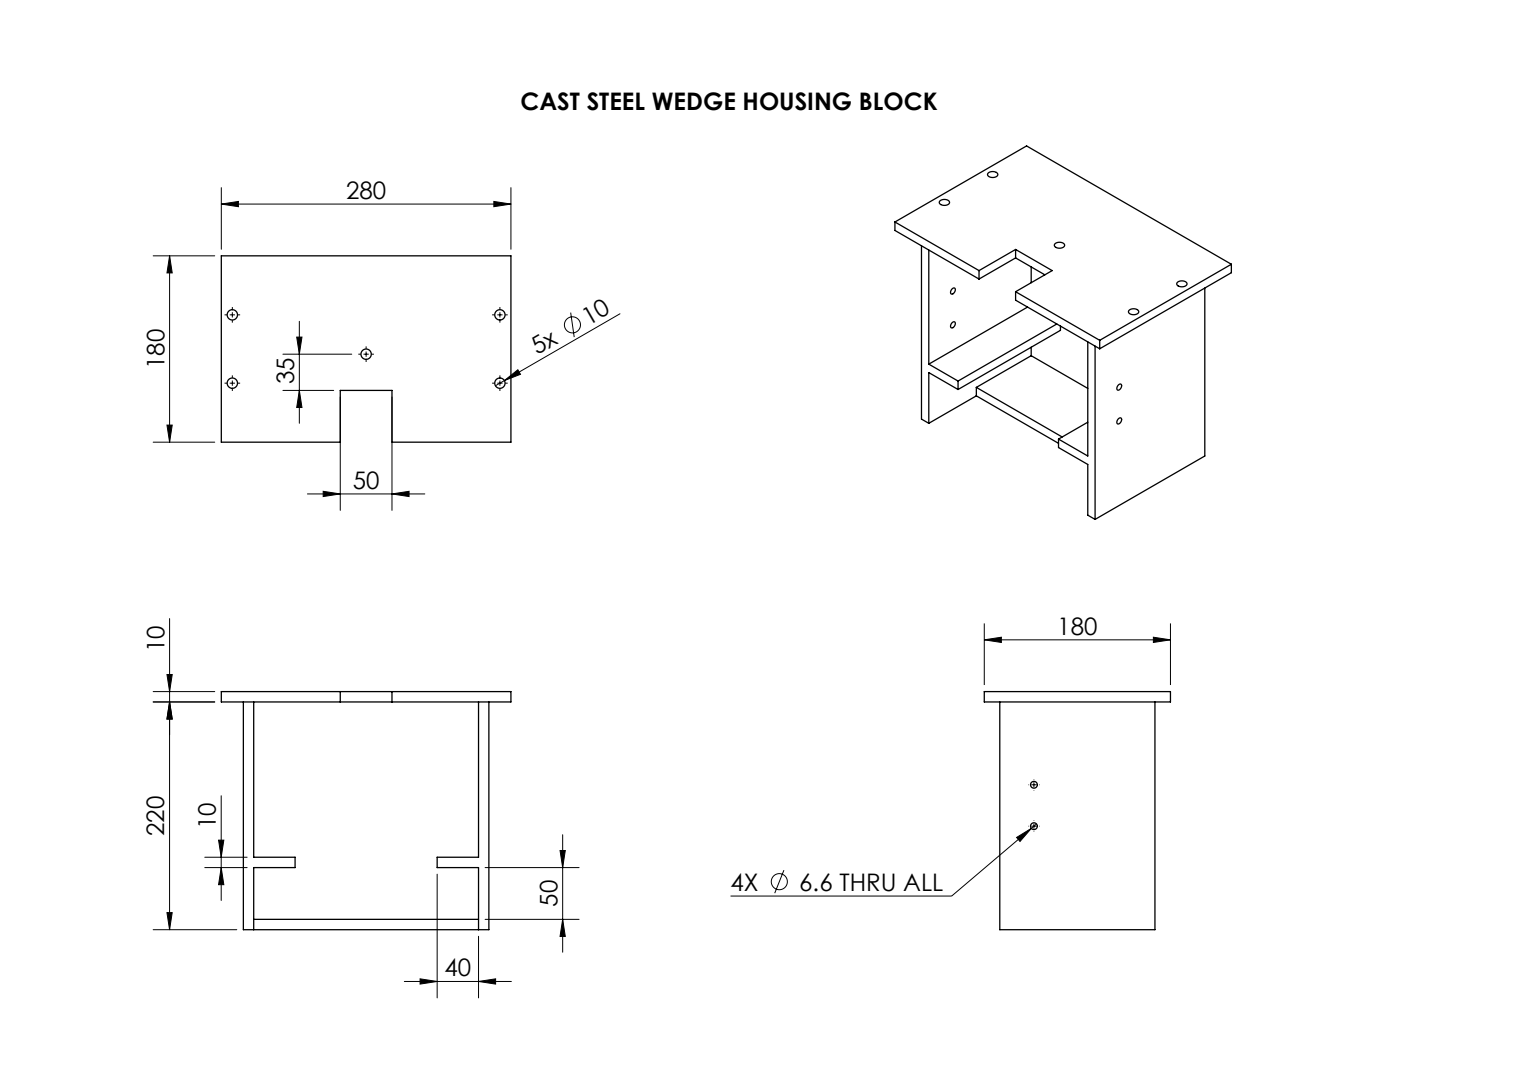
ISO-10303-21;
HEADER;
FILE_DESCRIPTION (('STEP AP214'),
    '1' );
FILE_NAME ('Cast Steel Wedge Housing Block.step',
    '2026-09-24T10:26:00',
    ( '' ),
    ( '' ),
    'SwSTEP 2.0',
    'SolidWorks 2026',
    '' );
FILE_SCHEMA (( 'AUTOMOTIVE_DESIGN' ));
ENDSEC;

DATA;
#1=VERTEX_POINT ( 'NONE', #3163 ) ;
#16=LINE ( 'NONE', #8451, #3074 ) ;
#26=LINE ( 'NONE', #9828, #8340 ) ;
#37=EDGE_CURVE ( 'NONE', #1523, #9034, #1990, .T. ) ;
#49=CARTESIAN_POINT ( 'NONE',  ( -129.3408537872145132, 199.5765550933606107, -75.00000000000001421 ) ) ;
#82=CARTESIAN_POINT ( 'NONE',  ( -108.6817075744281595, 69.57655509336026967, 0.000000000000000000 ) ) ;
#105=ORIENTED_EDGE ( 'NONE', *, *, #7029, .T. ) ;
#112=ORIENTED_EDGE ( 'NONE', *, *, #12518, .T. ) ;
#115=LINE ( 'NONE', #14321, #13122 ) ;
#130=EDGE_CURVE ( 'NONE', #3893, #6812, #6927, .T. ) ;
#149=LINE ( 'NONE', #2412, #13592 ) ;
#167=CARTESIAN_POINT ( 'NONE',  ( 0.000000000000000000, 0.000000000000000000, 0.000000000000000000 ) ) ;
#179=( NAMED_UNIT ( * ) PLANE_ANGLE_UNIT ( ) SI_UNIT ( $, .RADIAN. ) );
#185=ORIENTED_EDGE ( 'NONE', *, *, #3525, .T. ) ;
#186=DIRECTION ( 'NONE',  ( 0.000000000000000000, 0.000000000000000000, -1.000000000000000000 ) ) ;
#191=FACE_OUTER_BOUND ( 'NONE', #2606, .T. ) ;
#195=ADVANCED_FACE ( 'NONE', ( #8392 ), #5103, .F. ) ;
#215=LINE ( 'NONE', #3596, #1161 ) ;
#225=EDGE_CURVE ( 'NONE', #10568, #2459, #4887, .T. ) ;
#236=DIRECTION ( 'NONE',  ( 1.000000000000000000, -0.000000000000000000, -0.000000000000000000 ) ) ;
#237=AXIS2_PLACEMENT_3D ( 'NONE', #9091, #4649, #3762 ) ;
#243=DIRECTION ( 'NONE',  ( 1.000000000000000000, 1.723842398015259277E-15, 0.000000000000000000 ) ) ;
#250=PRESENTATION_STYLE_ASSIGNMENT (( #7854 ) ) ;
#252=LINE ( 'NONE', #13664, #5773 ) ;
#254=VERTEX_POINT ( 'NONE', #10524 ) ;
#256=ORIENTED_EDGE ( 'NONE', *, *, #409, .F. ) ;
#264=ADVANCED_FACE ( 'NONE', ( #14056 ), #3951, .T. ) ;
#268=CIRCLE ( 'NONE', #9369, 5.000000000000004441 ) ;
#275=FILL_AREA_STYLE_COLOUR ( '', #447 ) ;
#287=AXIS2_PLACEMENT_3D ( 'NONE', #9499, #13966, #10597 ) ;
#300=DIRECTION ( 'NONE',  ( -1.000000000000000000, -1.276920294826118092E-16, 0.000000000000000000 ) ) ;
#333=CARTESIAN_POINT ( 'NONE',  ( 108.6817075744280174, -30.42344490663958112, 33.00000000000002842 ) ) ;
#334=LINE ( 'NONE', #480, #12683 ) ;
#335=ORIENTED_EDGE ( 'NONE', *, *, #3874, .F. ) ;
#347=PRESENTATION_STYLE_ASSIGNMENT (( #11533 ) ) ;
#352=CARTESIAN_POINT ( 'NONE',  ( 25.00000000000000000, 189.5765550933606107, 47.99999999999998579 ) ) ;
#365=CARTESIAN_POINT ( 'NONE',  ( 129.3408537872138595, 189.5765550933606107, -4.000000000000019540 ) ) ;
#380=DIRECTION ( 'NONE',  ( 0.000000000000000000, 0.000000000000000000, -1.000000000000000000 ) ) ;
#393=ORIENTED_EDGE ( 'NONE', *, *, #4064, .F. ) ;
#408=VERTEX_POINT ( 'NONE', #8758 ) ;
#409=EDGE_CURVE ( 'NONE', #3034, #3463, #1002, .T. ) ;
#412=CARTESIAN_POINT ( 'NONE',  ( -140.0000000000003411, 189.5765550933606107, 47.99999999999998579 ) ) ;
#417=SURFACE_STYLE_FILL_AREA ( #8158 ) ;
#433=VERTEX_POINT ( 'NONE', #855 ) ;
#439=CARTESIAN_POINT ( 'NONE',  ( -108.6817075744280885, 39.57655509336044730, -117.0000000000000000 ) ) ;
#441=CARTESIAN_POINT ( 'NONE',  ( -108.6817075744282590, 189.5765550933606107, 33.00000000000002842 ) ) ;
#442=CARTESIAN_POINT ( 'NONE',  ( 139.9999999999996874, 199.5765550933606107, -132.0000000000000000 ) ) ;
#447=COLOUR_RGB ( '', 0.72549020, 0.75294118, 0.79215686) ;
#454=VECTOR ( 'NONE', #10609, 1000.000000000000000 ) ;
#456=ORIENTED_EDGE ( 'NONE', *, *, #10902, .F. ) ;
#463=DIRECTION ( 'NONE',  ( 1.000000000000000000, 1.723842398015259277E-15, -0.000000000000000000 ) ) ;
#468=CARTESIAN_POINT ( 'NONE',  ( -129.3408537872145132, 189.5765550933606107, -75.00000000000001421 ) ) ;
#470=CARTESIAN_POINT ( 'NONE',  ( -25.00000000000000000, 199.5765550933606107, 47.99999999999998579 ) ) ;
#476=VECTOR ( 'NONE', #6168, 1000.000000000000000 ) ;
#480=CARTESIAN_POINT ( 'NONE',  ( -118.6817075744281595, 69.57655509336025546, -3.299999999999976730 ) ) ;
#481=EDGE_LOOP ( 'NONE', ( #7301, #528 ) ) ;
#491=DIRECTION ( 'NONE',  ( -2.081668171172169499E-16, 0.000000000000000000, 1.000000000000000000 ) ) ;
#497=CARTESIAN_POINT ( 'NONE',  ( 129.3408537872138595, 199.5765550933606107, -13.99999999999999645 ) ) ;
#500=VECTOR ( 'NONE', #1584, 1000.000000000000000 ) ;
#505=CARTESIAN_POINT ( 'NONE',  ( -108.6817075744280174, -30.42344490663958112, 47.99999999999998579 ) ) ;
#506=ORIENTED_EDGE ( 'NONE', *, *, #6821, .T. ) ;
#528=ORIENTED_EDGE ( 'NONE', *, *, #1670, .T. ) ;
#532=( GEOMETRIC_REPRESENTATION_CONTEXT ( 3 ) GLOBAL_UNCERTAINTY_ASSIGNED_CONTEXT ( ( #5003 ) ) GLOBAL_UNIT_ASSIGNED_CONTEXT ( ( #13584, #179, #1134 ) ) REPRESENTATION_CONTEXT ( 'NONE', 'WORKASPACE' ) );
#537=FACE_OUTER_BOUND ( 'NONE', #8582, .T. ) ;
#539=DIRECTION ( 'NONE',  ( 0.000000000000000000, 0.000000000000000000, -1.000000000000000000 ) ) ;
#562=VERTEX_POINT ( 'NONE', #3500 ) ;
#570=CARTESIAN_POINT ( 'NONE',  ( -25.00000000000000000, -30.42444490663959300, 47.99999999999998579 ) ) ;
#574=CARTESIAN_POINT ( 'NONE',  ( -108.6817075744280174, -30.42344490663958112, 33.00000000000002842 ) ) ;
#577=ADVANCED_FACE ( 'NONE', ( #191 ), #8077, .F. ) ;
#582=PLANE ( 'NONE',  #287 ) ;
#597=ORIENTED_EDGE ( 'NONE', *, *, #130, .F. ) ;
#602=CARTESIAN_POINT ( 'NONE',  ( 108.6817075744280459, 189.5765550933606107, -106.9999999999999858 ) ) ;
#613=ORIENTED_EDGE ( 'NONE', *, *, #4304, .T. ) ;
#615=AXIS2_PLACEMENT_3D ( 'NONE', #11565, #1541, #13643 ) ;
#626=EDGE_LOOP ( 'NONE', ( #10160, #3816, #10628, #10696 ) ) ;
#631=CARTESIAN_POINT ( 'NONE',  ( -108.6817075744279748, 39.57655509336049704, -106.9999999999999858 ) ) ;
#636=CARTESIAN_POINT ( 'NONE',  ( -108.6817075744279748, 29.57655509336048993, -106.9999999999999858 ) ) ;
#644=CARTESIAN_POINT ( 'NONE',  ( -108.6817075744282448, 109.5765550933602839, -3.299999999999976730 ) ) ;
#663=VERTEX_POINT ( 'NONE', #11528 ) ;
#668=LINE ( 'NONE', #3960, #5178 ) ;
#675=CYLINDRICAL_SURFACE ( 'NONE', #9158, 4.999999999999976907 ) ;
#692=ORIENTED_EDGE ( 'NONE', *, *, #7072, .F. ) ;
#694=FACE_BOUND ( 'NONE', #11112, .T. ) ;
#701=ADVANCED_FACE ( 'NONE', ( #4946 ), #3933, .T. ) ;
#714=CARTESIAN_POINT ( 'NONE',  ( -88.22284556172397174, 29.57655509336047572, -106.9999999999999858 ) ) ;
#716=VERTEX_POINT ( 'NONE', #7054 ) ;
#722=DIRECTION ( 'NONE',  ( 0.000000000000000000, 0.000000000000000000, 1.000000000000000000 ) ) ;
#731=LINE ( 'NONE', #8625, #5410 ) ;
#737=ORIENTED_EDGE ( 'NONE', *, *, #6925, .T. ) ;
#767=LINE ( 'NONE', #826, #476 ) ;
#768=VERTEX_POINT ( 'NONE', #5023 ) ;
#779=LINE ( 'NONE', #3128, #5895 ) ;
#784=EDGE_CURVE ( 'NONE', #562, #2174, #4802, .T. ) ;
#794=ORIENTED_EDGE ( 'NONE', *, *, #7642, .F. ) ;
#795=DIRECTION ( 'NONE',  ( 1.000000000000000000, 0.000000000000000000, 0.000000000000000000 ) ) ;
#807=DIRECTION ( 'NONE',  ( 0.000000000000000000, 0.000000000000000000, -1.000000000000000000 ) ) ;
#810=ORIENTED_EDGE ( 'NONE', *, *, #14188, .T. ) ;
#811=ADVANCED_FACE ( 'NONE', ( #2088 ), #4307, .T. ) ;
#826=CARTESIAN_POINT ( 'NONE',  ( 68.68170757442801744, 39.57655509336063915, -117.0000000000000000 ) ) ;
#835=CARTESIAN_POINT ( 'NONE',  ( -68.68170757442808849, 39.57655509336051836, 33.00000000000002842 ) ) ;
#847=FACE_OUTER_BOUND ( 'NONE', #5857, .T. ) ;
#850=VECTOR ( 'NONE', #2149, 1000.000000000000000 ) ;
#854=ORIENTED_EDGE ( 'NONE', *, *, #1139, .T. ) ;
#855=CARTESIAN_POINT ( 'NONE',  ( -108.6817075744282448, 109.5765550933602839, 3.299999999999976730 ) ) ;
#875=CARTESIAN_POINT ( 'NONE',  ( 25.00000000000000000, 189.5765550933605539, 47.99999999999998579 ) ) ;
#887=CARTESIAN_POINT ( 'NONE',  ( -1.080113255961760282E-14, -20.42344490663947809, -32.00000000000002842 ) ) ;
#888=DIRECTION ( 'NONE',  ( 0.000000000000000000, 1.000000000000000000, 0.000000000000000000 ) ) ;
#898=EDGE_CURVE ( 'NONE', #5390, #9318, #7561, .T. ) ;
#900=CARTESIAN_POINT ( 'NONE',  ( 25.00000000000000000, -30.42444490663959300, 47.99999999999998579 ) ) ;
#919=EDGE_LOOP ( 'NONE', ( #5334, #5364 ) ) ;
#925=DIRECTION ( 'NONE',  ( 0.000000000000000000, 1.000000000000000000, 0.000000000000000000 ) ) ;
#935=EDGE_LOOP ( 'NONE', ( #9842, #13555 ) ) ;
#960=DIRECTION ( 'NONE',  ( 1.000000000000000000, 0.000000000000000000, -0.000000000000000000 ) ) ;
#963=ADVANCED_FACE ( 'NONE', ( #6894 ), #8876, .T. ) ;
#972=DIRECTION ( 'NONE',  ( 0.000000000000000000, 0.000000000000000000, -1.000000000000000000 ) ) ;
#977=LINE ( 'NONE', #3056, #12454 ) ;
#980=ORIENTED_EDGE ( 'NONE', *, *, #12175, .T. ) ;
#997=CARTESIAN_POINT ( 'NONE',  ( 25.00000000000000000, -30.42444490663959300, 47.99999999999998579 ) ) ;
#998=EDGE_LOOP ( 'NONE', ( #1138, #3336, #3674, #9765 ) ) ;
#999=EDGE_CURVE ( 'NONE', #9323, #10543, #7783, .T. ) ;
#1002=LINE ( 'NONE', #14406, #5232 ) ;
#1015=ADVANCED_FACE ( 'NONE', ( #10127 ), #9015, .F. ) ;
#1047=DIRECTION ( 'NONE',  ( 0.000000000000000000, 0.000000000000000000, 1.000000000000000000 ) ) ;
#1066=LINE ( 'NONE', #10874, #1839 ) ;
#1067=ORIENTED_EDGE ( 'NONE', *, *, #2065, .F. ) ;
#1072=EDGE_LOOP ( 'NONE', ( #5271, #2451, #3300, #1091 ) ) ;
#1076=EDGE_LOOP ( 'NONE', ( #10467, #5477, #3567, #7124 ) ) ;
#1091=ORIENTED_EDGE ( 'NONE', *, *, #9473, .F. ) ;
#1096=CARTESIAN_POINT ( 'NONE',  ( -129.3408537872145132, 199.5765550933606107, -70.00000000000000000 ) ) ;
#1097=ORIENTED_EDGE ( 'NONE', *, *, #7571, .T. ) ;
#1115=LINE ( 'NONE', #6668, #10498 ) ;
#1116=AXIS2_PLACEMENT_3D ( 'NONE', #1564, #3493, #4656 ) ;
#1132=DIRECTION ( 'NONE',  ( 0.000000000000000000, 0.000000000000000000, 1.000000000000000000 ) ) ;
#1134=( NAMED_UNIT ( * ) SI_UNIT ( $, .STERADIAN. ) SOLID_ANGLE_UNIT ( ) );
#1138=ORIENTED_EDGE ( 'NONE', *, *, #8326, .T. ) ;
#1139=EDGE_CURVE ( 'NONE', #9318, #5054, #10407, .T. ) ;
#1161=VECTOR ( 'NONE', #2481, 1000.000000000000000 ) ;
#1185=EDGE_CURVE ( 'NONE', #3592, #433, #14284, .T. ) ;
#1189=EDGE_CURVE ( 'NONE', #3592, #5863, #6306, .T. ) ;
#1204=DIRECTION ( 'NONE',  ( 0.000000000000000000, 0.000000000000000000, 1.000000000000000000 ) ) ;
#1206=CARTESIAN_POINT ( 'NONE',  ( 108.6817075744280459, 189.5765550933606107, 33.00000000000002842 ) ) ;
#1219=VERTEX_POINT ( 'NONE', #3111 ) ;
#1234=EDGE_LOOP ( 'NONE', ( #7527, #4857, #14209, #14238 ) ) ;
#1259=DIRECTION ( 'NONE',  ( 0.000000000000000000, 0.000000000000000000, 1.000000000000000000 ) ) ;
#1272=DIRECTION ( 'NONE',  ( 0.000000000000000000, 0.000000000000000000, 1.000000000000000000 ) ) ;
#1282=EDGE_CURVE ( 'NONE', #4218, #7189, #7608, .T. ) ;
#1294=CARTESIAN_POINT ( 'NONE',  ( 139.9999999999996874, 189.5765550933606107, -132.0000000000000000 ) ) ;
#1308=LINE ( 'NONE', #5757, #1678 ) ;
#1319=DIRECTION ( 'NONE',  ( 0.000000000000000000, 1.000000000000000000, -0.000000000000000000 ) ) ;
#1320=VERTEX_POINT ( 'NONE', #5501 ) ;
#1324=CARTESIAN_POINT ( 'NONE',  ( 118.6817075744280316, 109.5765550933604828, 0.000000000000000000 ) ) ;
#1325=VECTOR ( 'NONE', #14394, 1000.000000000000000 ) ;
#1330=EDGE_LOOP ( 'NONE', ( #14150, #4446, #3501, #2087, #3645, #980, #2647, #10197 ) ) ;
#1344=VERTEX_POINT ( 'NONE', #12164 ) ;
#1360=AXIS2_PLACEMENT_3D ( 'NONE', #49, #11157, #14398 ) ;
#1365=CARTESIAN_POINT ( 'NONE',  ( -129.3408537872145132, 189.5765550933606107, -70.00000000000000000 ) ) ;
#1380=DIRECTION ( 'NONE',  ( 0.000000000000000000, 1.000000000000000000, 0.000000000000000000 ) ) ;
#1396=VECTOR ( 'NONE', #6858, 1000.000000000000000 ) ;
#1397=LINE ( 'NONE', #2579, #11974 ) ;
#1416=ORIENTED_EDGE ( 'NONE', *, *, #13645, .F. ) ;
#1417=CARTESIAN_POINT ( 'NONE',  ( -140.0000000000003411, 189.5765550933606107, 47.99999999999998579 ) ) ;
#1426=ORIENTED_EDGE ( 'NONE', *, *, #3621, .T. ) ;
#1432=DIRECTION ( 'NONE',  ( -1.000000000000000000, -8.619211990076296383E-16, 0.000000000000000000 ) ) ;
#1433=CARTESIAN_POINT ( 'NONE',  ( 118.6817075744280316, 109.5765550933604828, 0.000000000000000000 ) ) ;
#1442=FACE_OUTER_BOUND ( 'NONE', #10048, .T. ) ;
#1447=ORIENTED_EDGE ( 'NONE', *, *, #2115, .T. ) ;
#1451=CIRCLE ( 'NONE', #3083, 3.299999999999969624 ) ;
#1469=EDGE_CURVE ( 'NONE', #3034, #3917, #16, .T. ) ;
#1474=DIRECTION ( 'NONE',  ( 1.000000000000000000, 0.000000000000000000, -0.000000000000000000 ) ) ;
#1477=VERTEX_POINT ( 'NONE', #13348 ) ;
#1485=DIRECTION ( 'NONE',  ( 0.000000000000000000, 0.000000000000000000, -1.000000000000000000 ) ) ;
#1496=ORIENTED_EDGE ( 'NONE', *, *, #3852, .F. ) ;
#1510=DIRECTION ( 'NONE',  ( 1.000000000000000000, 0.000000000000000000, -0.000000000000000000 ) ) ;
#1519=PLANE ( 'NONE',  #4004 ) ;
#1523=VERTEX_POINT ( 'NONE', #14370 ) ;
#1536=CARTESIAN_POINT ( 'NONE',  ( -118.6817075744282306, 109.5765550933602839, 3.299999999999983391 ) ) ;
#1538=EDGE_LOOP ( 'NONE', ( #4094, #2861 ) ) ;
#1541=DIRECTION ( 'NONE',  ( 1.000000000000000000, 1.913084959030911013E-15, 0.000000000000000000 ) ) ;
#1551=VERTEX_POINT ( 'NONE', #13204 ) ;
#1564=CARTESIAN_POINT ( 'NONE',  ( -108.6817075744281595, 69.57655509336026967, 0.000000000000000000 ) ) ;
#1575=CARTESIAN_POINT ( 'NONE',  ( 139.9999999999996874, 199.5765550933606107, 47.99999999999998579 ) ) ;
#1579=EDGE_CURVE ( 'NONE', #1934, #3640, #10326, .T. ) ;
#1584=DIRECTION ( 'NONE',  ( -1.321694076934709169E-16, 1.000000000000000000, -0.000000000000000000 ) ) ;
#1636=DIRECTION ( 'NONE',  ( 0.000000000000000000, -1.000000000000000000, -0.000000000000000000 ) ) ;
#1643=DIRECTION ( 'NONE',  ( 0.000000000000000000, 1.000000000000000000, 0.000000000000000000 ) ) ;
#1659=SURFACE_SIDE_STYLE ('',( #417 ) ) ;
#1667=FACE_BOUND ( 'NONE', #4349, .T. ) ;
#1668=AXIS2_PLACEMENT_3D ( 'NONE', #1417, #2595, #7041 ) ;
#1670=EDGE_CURVE ( 'NONE', #408, #8822, #268, .T. ) ;
#1678=VECTOR ( 'NONE', #13260, 1000.000000000000000 ) ;
#1683=PLANE ( 'NONE',  #4495 ) ;
#1686=LINE ( 'NONE', #602, #7972 ) ;
#1695=ORIENTED_EDGE ( 'NONE', *, *, #1670, .F. ) ;
#1697=LINE ( 'NONE', #10547, #5430 ) ;
#1699=COLOUR_RGB ( '', 0.72549020, 0.75294118, 0.79215686) ;
#1747=DIRECTION ( 'NONE',  ( 1.000000000000000000, -0.000000000000000000, -0.000000000000000000 ) ) ;
#1759=DIRECTION ( 'NONE',  ( -0.000000000000000000, 1.000000000000000000, -0.000000000000000000 ) ) ;
#1769=ORIENTED_EDGE ( 'NONE', *, *, #8326, .F. ) ;
#1779=VECTOR ( 'NONE', #960, 1000.000000000000000 ) ;
#1785=DIRECTION ( 'NONE',  ( 0.000000000000000000, -1.000000000000000000, 0.000000000000000000 ) ) ;
#1790=DIRECTION ( 'NONE',  ( 1.000000000000000000, 0.000000000000000000, -0.000000000000000000 ) ) ;
#1812=CARTESIAN_POINT ( 'NONE',  ( 129.3408537872138595, 189.5765550933606107, -13.99999999999999645 ) ) ;
#1818=VECTOR ( 'NONE', #11234, 1000.000000000000000 ) ;
#1823=ORIENTED_EDGE ( 'NONE', *, *, #7239, .F. ) ;
#1824=FACE_OUTER_BOUND ( 'NONE', #8561, .T. ) ;
#1829=DIRECTION ( 'NONE',  ( -1.000000000000000000, 1.892425610156516875E-16, 0.000000000000000000 ) ) ;
#1839=VECTOR ( 'NONE', #13298, 1000.000000000000000 ) ;
#1858=FACE_OUTER_BOUND ( 'NONE', #1072, .T. ) ;
#1876=DIRECTION ( 'NONE',  ( 1.000000000000000000, 0.000000000000000000, 0.000000000000000000 ) ) ;
#1894=ORIENTED_EDGE ( 'NONE', *, *, #6821, .F. ) ;
#1895=ORIENTED_EDGE ( 'NONE', *, *, #1579, .F. ) ;
#1903=FACE_OUTER_BOUND ( 'NONE', #10336, .T. ) ;
#1914=CIRCLE ( 'NONE', #11959, 4.999999999999976907 ) ;
#1930=VECTOR ( 'NONE', #5761, 1000.000000000000000 ) ;
#1933=CARTESIAN_POINT ( 'NONE',  ( -68.68170757442787533, -83.66032599071911591, -106.9999999999999858 ) ) ;
#1934=VERTEX_POINT ( 'NONE', #365 ) ;
#1941=CYLINDRICAL_SURFACE ( 'NONE', #12796, 5.000000000000004441 ) ;
#1943=CIRCLE ( 'NONE', #8007, 3.299999999999983391 ) ;
#1955=CARTESIAN_POINT ( 'NONE',  ( -118.6817075744282306, 109.5765550933602697, -3.299999999999983391 ) ) ;
#1956=VECTOR ( 'NONE', #1485, 1000.000000000000000 ) ;
#1958=CARTESIAN_POINT ( 'NONE',  ( -24.99999999999998934, -30.42444490663959300, -2.000000000000001776 ) ) ;
#1962=EDGE_CURVE ( 'NONE', #13737, #768, #215, .T. ) ;
#1963=DIRECTION ( 'NONE',  ( 0.000000000000000000, -0.000000000000000000, -1.000000000000000000 ) ) ;
#1986=ORIENTED_EDGE ( 'NONE', *, *, #37, .F. ) ;
#1990=CIRCLE ( 'NONE', #7575, 3.299999999999969624 ) ;
#1993=ORIENTED_EDGE ( 'NONE', *, *, #13450, .F. ) ;
#2004=PLANE ( 'NONE',  #4907 ) ;
#2025=CARTESIAN_POINT ( 'NONE',  ( -140.0000000000003411, 189.5765550933606107, -132.0000000000000000 ) ) ;
#2036=CARTESIAN_POINT ( 'NONE',  ( 118.6817075744280316, 69.57655509336046862, 3.299999999999982947 ) ) ;
#2049=VECTOR ( 'NONE', #4297, 1000.000000000000000 ) ;
#2051=CIRCLE ( 'NONE', #8821, 4.999999999999988454 ) ;
#2054=DIRECTION ( 'NONE',  ( -1.000000000000000000, 0.000000000000000000, 0.000000000000000000 ) ) ;
#2058=AXIS2_PLACEMENT_3D ( 'NONE', #13499, #3616, #3752 ) ;
#2065=EDGE_CURVE ( 'NONE', #2858, #254, #4035, .T. ) ;
#2068=DIRECTION ( 'NONE',  ( 0.000000000000000000, 1.000000000000000000, -0.000000000000000000 ) ) ;
#2070=EDGE_CURVE ( 'NONE', #9480, #12696, #4893, .T. ) ;
#2073=DIRECTION ( 'NONE',  ( 0.000000000000000000, -0.000000000000000000, -1.000000000000000000 ) ) ;
#2078=LINE ( 'NONE', #3409, #8110 ) ;
#2082=DIRECTION ( 'NONE',  ( 1.000000000000000000, 8.619211990076297369E-16, 0.000000000000000000 ) ) ;
#2087=ORIENTED_EDGE ( 'NONE', *, *, #3724, .T. ) ;
#2088=FACE_OUTER_BOUND ( 'NONE', #13599, .T. ) ;
#2092=DIRECTION ( 'NONE',  ( -1.723842398015259277E-15, 1.000000000000000000, 0.000000000000000000 ) ) ;
#2095=ORIENTED_EDGE ( 'NONE', *, *, #2070, .F. ) ;
#2096=CARTESIAN_POINT ( 'NONE',  ( -118.6817075744279748, -20.42344490663959178, 33.00000000000002842 ) ) ;
#2115=EDGE_CURVE ( 'NONE', #2459, #5279, #11552, .T. ) ;
#2121=ORIENTED_EDGE ( 'NONE', *, *, #11840, .F. ) ;
#2124=VECTOR ( 'NONE', #8164, 1000.000000000000000 ) ;
#2136=EDGE_CURVE ( 'NONE', #8708, #663, #6209, .T. ) ;
#2149=DIRECTION ( 'NONE',  ( 0.000000000000000000, 0.000000000000000000, 1.000000000000000000 ) ) ;
#2161=VECTOR ( 'NONE', #12396, 1000.000000000000000 ) ;
#2162=MECHANICAL_DESIGN_GEOMETRIC_PRESENTATION_REPRESENTATION('',(#2391),#2881);
#2166=ORIENTED_EDGE ( 'NONE', *, *, #12229, .T. ) ;
#2174=VERTEX_POINT ( 'NONE', #7145 ) ;
#2176=LINE ( 'NONE', #2096, #3085 ) ;
#2177=EDGE_CURVE ( 'NONE', #5014, #2858, #3957, .T. ) ;
#2182=ORIENTED_EDGE ( 'NONE', *, *, #3874, .T. ) ;
#2226=DIRECTION ( 'NONE',  ( 0.000000000000000000, 1.000000000000000000, 0.000000000000000000 ) ) ;
#2233=ORIENTED_EDGE ( 'NONE', *, *, #7103, .F. ) ;
#2309=ORIENTED_EDGE ( 'NONE', *, *, #14188, .F. ) ;
#2310=LINE ( 'NONE', #2025, #3690 ) ;
#2335=EDGE_LOOP ( 'NONE', ( #2309, #9256 ) ) ;
#2350=DIRECTION ( 'NONE',  ( -0.000000000000000000, 1.000000000000000000, -0.000000000000000000 ) ) ;
#2369=EDGE_LOOP ( 'NONE', ( #9647, #9703, #2381, #4239, #3780, #506 ) ) ;
#2381=ORIENTED_EDGE ( 'NONE', *, *, #2115, .F. ) ;
#2391=STYLED_ITEM ( 'NONE', ( #250 ), #14323 ) ;
#2410=DIRECTION ( 'NONE',  ( -0.000000000000000000, -0.000000000000000000, 1.000000000000000000 ) ) ;
#2412=CARTESIAN_POINT ( 'NONE',  ( 118.6817075744280174, -20.42344490663938927, 33.00000000000002842 ) ) ;
#2429=DIRECTION ( 'NONE',  ( 0.000000000000000000, 1.000000000000000000, 0.000000000000000000 ) ) ;
#2436=CLOSED_SHELL ( 'NONE', ( #7622, #13352, #7363, #5558, #4052, #5478, #8462, #6175, #12674, #5272, #963, #11640, #12561, #4775, #9859, #8044, #701, #5129, #7603, #10411, #5256, #811, #12606, #7549, #577, #12763, #2611, #6091, #4267, #9409, #7704, #10797, #9868, #264, #11833, #12856, #10203, #12636, #4124, #8382, #10124, #11221, #3466, #1015, #8733, #8910, #195 ) ) ;
#2438=CARTESIAN_POINT ( 'NONE',  ( -140.0000000000003411, 199.5765550933606107, -132.0000000000000000 ) ) ;
#2449=VECTOR ( 'NONE', #13472, 1000.000000000000000 ) ;
#2451=ORIENTED_EDGE ( 'NONE', *, *, #10501, .T. ) ;
#2457=AXIS2_PLACEMENT_3D ( 'NONE', #2670, #1636, #12530 ) ;
#2459=VERTEX_POINT ( 'NONE', #574 ) ;
#2464=EDGE_CURVE ( 'NONE', #2174, #9318, #9566, .T. ) ;
#2467=DIRECTION ( 'NONE',  ( -0.000000000000000000, 0.000000000000000000, -1.000000000000000000 ) ) ;
#2477=CARTESIAN_POINT ( 'NONE',  ( 118.6817075744280316, 69.57655509336046862, -3.299999999999976730 ) ) ;
#2478=EDGE_LOOP ( 'NONE', ( #4965, #2705, #11804, #1067 ) ) ;
#2481=DIRECTION ( 'NONE',  ( 1.000000000000000000, 0.000000000000000000, 0.000000000000000000 ) ) ;
#2502=FACE_BOUND ( 'NONE', #6506, .T. ) ;
#2504=VERTEX_POINT ( 'NONE', #3867 ) ;
#2507=PRODUCT_DEFINITION_SHAPE ( 'NONE', 'NONE',  #6941 ) ;
#2510=DIRECTION ( 'NONE',  ( 1.000000000000000000, 8.619211990076297369E-16, 0.000000000000000000 ) ) ;
#2511=VECTOR ( 'NONE', #3568, 1000.000000000000000 ) ;
#2521=ORIENTED_EDGE ( 'NONE', *, *, #9187, .T. ) ;
#2560=DIRECTION ( 'NONE',  ( 0.000000000000000000, 0.000000000000000000, -1.000000000000000000 ) ) ;
#2562=LINE ( 'NONE', #13698, #6339 ) ;
#2573=EDGE_CURVE ( 'NONE', #14451, #716, #9337, .T. ) ;
#2579=CARTESIAN_POINT ( 'NONE',  ( 68.68170757442801744, 29.57655509336062849, -117.0000000000000000 ) ) ;
#2595=DIRECTION ( 'NONE',  ( 0.000000000000000000, 0.000000000000000000, 1.000000000000000000 ) ) ;
#2606=EDGE_LOOP ( 'NONE', ( #14177, #5927, #335, #11394, #3892, #3979, #10224, #1426 ) ) ;
#2611=ADVANCED_FACE ( 'NONE', ( #4378 ), #4237, .F. ) ;
#2614=PLANE ( 'NONE',  #11399 ) ;
#2615=AXIS2_PLACEMENT_3D ( 'NONE', #4418, #12371, #7671 ) ;
#2617=LINE ( 'NONE', #1294, #3303 ) ;
#2619=CARTESIAN_POINT ( 'NONE',  ( 108.6817075744280174, -20.42344490663938572, 33.00000000000002842 ) ) ;
#2634=CARTESIAN_POINT ( 'NONE',  ( 88.22284556172391490, 29.57655509336062849, 33.00000000000002842 ) ) ;
#2647=ORIENTED_EDGE ( 'NONE', *, *, #4064, .T. ) ;
#2649=ORIENTED_EDGE ( 'NONE', *, *, #11568, .F. ) ;
#2658=ORIENTED_EDGE ( 'NONE', *, *, #12379, .T. ) ;
#2670=CARTESIAN_POINT ( 'NONE',  ( 118.6817075744280601, 199.5765550933606107, 33.00000000000002842 ) ) ;
#2674=CARTESIAN_POINT ( 'NONE',  ( 118.6817075744280174, -30.42344490663937506, 33.00000000000002842 ) ) ;
#2687=VERTEX_POINT ( 'NONE', #7714 ) ;
#2699=CARTESIAN_POINT ( 'NONE',  ( 68.68170757442801744, -83.66032599071898801, -117.0000000000000000 ) ) ;
#2705=ORIENTED_EDGE ( 'NONE', *, *, #3724, .F. ) ;
#2716=EDGE_CURVE ( 'NONE', #2174, #4711, #11982, .T. ) ;
#2719=LINE ( 'NONE', #13632, #9855 ) ;
#2722=ORIENTED_EDGE ( 'NONE', *, *, #12323, .F. ) ;
#2730=ORIENTED_EDGE ( 'NONE', *, *, #8142, .T. ) ;
#2734=CIRCLE ( 'NONE', #10898, 3.299999999999983391 ) ;
#2741=FACE_BOUND ( 'NONE', #3207, .T. ) ;
#2747=AXIS2_PLACEMENT_3D ( 'NONE', #5724, #10200, #186 ) ;
#2752=LINE ( 'NONE', #2829, #5547 ) ;
#2774=CARTESIAN_POINT ( 'NONE',  ( 0.000000000000000000, 0.000000000000000000, -106.9999999999999858 ) ) ;
#2780=ORIENTED_EDGE ( 'NONE', *, *, #12032, .F. ) ;
#2782=VERTEX_POINT ( 'NONE', #1206 ) ;
#2788=DIRECTION ( 'NONE',  ( 0.000000000000000000, 0.000000000000000000, 1.000000000000000000 ) ) ;
#2792=DIRECTION ( 'NONE',  ( -1.276920294826117846E-16, 0.000000000000000000, -1.000000000000000000 ) ) ;
#2794=DIRECTION ( 'NONE',  ( 0.000000000000000000, 0.000000000000000000, -1.000000000000000000 ) ) ;
#2795=CARTESIAN_POINT ( 'NONE',  ( -68.68170757442808849, 39.57655509336051836, -117.0000000000000000 ) ) ;
#2813=AXIS2_PLACEMENT_3D ( 'NONE', #7440, #925, #13239 ) ;
#2828=CIRCLE ( 'NONE', #3522, 3.299999999999983391 ) ;
#2829=CARTESIAN_POINT ( 'NONE',  ( -129.3408537872145132, 189.5765550933606107, -70.00000000000000000 ) ) ;
#2858=VERTEX_POINT ( 'NONE', #631 ) ;
#2861=ORIENTED_EDGE ( 'NONE', *, *, #7993, .T. ) ;
#2864=CARTESIAN_POINT ( 'NONE',  ( -88.22284556172398595, 39.57655509336048283, -106.9999999999999858 ) ) ;
#2872=CIRCLE ( 'NONE', #7287, 3.299999999999983391 ) ;
#2878=ORIENTED_EDGE ( 'NONE', *, *, #8871, .T. ) ;
#2881=( GEOMETRIC_REPRESENTATION_CONTEXT ( 3 ) GLOBAL_UNCERTAINTY_ASSIGNED_CONTEXT ( ( #13058 ) ) GLOBAL_UNIT_ASSIGNED_CONTEXT ( ( #10642, #12755, #3849 ) ) REPRESENTATION_CONTEXT ( 'NONE', 'WORKASPACE' ) );
#2891=DIRECTION ( 'NONE',  ( 0.000000000000000000, -1.000000000000000000, 0.000000000000000000 ) ) ;
#2896=FACE_OUTER_BOUND ( 'NONE', #5590, .T. ) ;
#2900=FACE_OUTER_BOUND ( 'NONE', #11574, .T. ) ;
#2931=PLANE ( 'NONE',  #7167 ) ;
#2960=ORIENTED_EDGE ( 'NONE', *, *, #7391, .T. ) ;
#2967=EDGE_LOOP ( 'NONE', ( #456, #7975, #11692, #11861 ) ) ;
#3001=APPLICATION_CONTEXT ( 'automotive_design' ) ;
#3019=DIRECTION ( 'NONE',  ( 0.000000000000000000, 0.000000000000000000, 1.000000000000000000 ) ) ;
#3034=VERTEX_POINT ( 'NONE', #10023 ) ;
#3042=CARTESIAN_POINT ( 'NONE',  ( -118.6817075744281595, 69.57655509336026967, 3.299999999999982947 ) ) ;
#3044=EDGE_LOOP ( 'NONE', ( #7104, #6788, #3440, #2095 ) ) ;
#3047=VECTOR ( 'NONE', #7306, 1000.000000000000000 ) ;
#3049=EDGE_LOOP ( 'NONE', ( #7279, #7569, #10044, #185 ) ) ;
#3051=DIRECTION ( 'NONE',  ( 0.000000000000000000, 0.000000000000000000, 1.000000000000000000 ) ) ;
#3053=VECTOR ( 'NONE', #11999, 1000.000000000000000 ) ;
#3056=CARTESIAN_POINT ( 'NONE',  ( 139.9999999999996874, 199.5765550933606107, 47.99999999999998579 ) ) ;
#3059=DIRECTION ( 'NONE',  ( -1.000000000000000000, 0.000000000000000000, 1.387778780781446415E-16 ) ) ;
#3073=EDGE_LOOP ( 'NONE', ( #9571, #1894, #9487, #3953 ) ) ;
#3074=VECTOR ( 'NONE', #9897, 1000.000000000000000 ) ;
#3075=ORIENTED_EDGE ( 'NONE', *, *, #14001, .T. ) ;
#3080=DIRECTION ( 'NONE',  ( -1.000000000000000000, -1.723842398015259277E-15, 0.000000000000000000 ) ) ;
#3083=AXIS2_PLACEMENT_3D ( 'NONE', #5415, #13414, #12230 ) ;
#3085=VECTOR ( 'NONE', #9927, 1000.000000000000000 ) ;
#3111=CARTESIAN_POINT ( 'NONE',  ( 129.3408537872138595, 189.5765550933606107, -80.00000000000002842 ) ) ;
#3128=CARTESIAN_POINT ( 'NONE',  ( 6.118061346828462449E-15, -30.42344490663947809, -117.0000000000000000 ) ) ;
#3129=ORIENTED_EDGE ( 'NONE', *, *, #10296, .F. ) ;
#3134=VECTOR ( 'NONE', #243, 1000.000000000000000 ) ;
#3143=DIRECTION ( 'NONE',  ( -1.000000000000000000, -0.000000000000000000, -0.000000000000000000 ) ) ;
#3150=CYLINDRICAL_SURFACE ( 'NONE', #6770, 3.299999999999976730 ) ;
#3153=CARTESIAN_POINT ( 'NONE',  ( 108.6817075744280459, 109.5765550933604828, -3.299999999999976730 ) ) ;
#3163=CARTESIAN_POINT ( 'NONE',  ( 129.3408537872138595, 189.5765550933606107, -69.99999999999998579 ) ) ;
#3168=LINE ( 'NONE', #13195, #7244 ) ;
#3179=LINE ( 'NONE', #8860, #850 ) ;
#3199=FACE_OUTER_BOUND ( 'NONE', #14336, .T. ) ;
#3206=VECTOR ( 'NONE', #10561, 1000.000000000000000 ) ;
#3207=EDGE_LOOP ( 'NONE', ( #7908, #5778 ) ) ;
#3208=ORIENTED_EDGE ( 'NONE', *, *, #11066, .T. ) ;
#3213=EDGE_CURVE ( 'NONE', #716, #5014, #4141, .T. ) ;
#3226=DIRECTION ( 'NONE',  ( -1.000000000000000000, 1.892425610156516875E-16, 0.000000000000000000 ) ) ;
#3241=CARTESIAN_POINT ( 'NONE',  ( 108.6817075744280316, -30.42344490663958112, -32.00000000000002842 ) ) ;
#3250=CARTESIAN_POINT ( 'NONE',  ( 139.9999999999996874, 189.5765550933606107, 47.99999999999998579 ) ) ;
#3251=EDGE_CURVE ( 'NONE', #14451, #5279, #3179, .T. ) ;
#3260=EDGE_CURVE ( 'NONE', #6812, #6602, #2734, .T. ) ;
#3261=DIRECTION ( 'NONE',  ( -1.000000000000000000, -0.000000000000000000, -0.000000000000000000 ) ) ;
#3300=ORIENTED_EDGE ( 'NONE', *, *, #12821, .T. ) ;
#3303=VECTOR ( 'NONE', #3585, 1000.000000000000000 ) ;
#3316=EDGE_LOOP ( 'NONE', ( #4766, #10357, #7339, #6949 ) ) ;
#3328=DIRECTION ( 'NONE',  ( 0.000000000000000000, 0.000000000000000000, -1.000000000000000000 ) ) ;
#3336=ORIENTED_EDGE ( 'NONE', *, *, #1469, .T. ) ;
#3346=EDGE_CURVE ( 'NONE', #716, #14013, #7689, .T. ) ;
#3355=ORIENTED_EDGE ( 'NONE', *, *, #2716, .F. ) ;
#3363=CARTESIAN_POINT ( 'NONE',  ( 6.118061346828462449E-15, -30.42344490663947809, 33.00000000000002842 ) ) ;
#3382=ORIENTED_EDGE ( 'NONE', *, *, #4255, .F. ) ;
#3393=VERTEX_POINT ( 'NONE', #3250 ) ;
#3400=CYLINDRICAL_SURFACE ( 'NONE', #14432, 4.999999999999988454 ) ;
#3403=DIRECTION ( 'NONE',  ( 1.000000000000000000, -0.000000000000000000, -0.000000000000000000 ) ) ;
#3409=CARTESIAN_POINT ( 'NONE',  ( 139.9999999999996874, 189.5765550933606107, 47.99999999999998579 ) ) ;
#3414=DIRECTION ( 'NONE',  ( 0.000000000000000000, 1.000000000000000000, -0.000000000000000000 ) ) ;
#3415=LINE ( 'NONE', #7626, #2161 ) ;
#3440=ORIENTED_EDGE ( 'NONE', *, *, #4370, .T. ) ;
#3463=VERTEX_POINT ( 'NONE', #1575 ) ;
#3464=FACE_OUTER_BOUND ( 'NONE', #12416, .T. ) ;
#3466=ADVANCED_FACE ( 'NONE', ( #6104 ), #8078, .F. ) ;
#3469=AXIS2_PLACEMENT_3D ( 'NONE', #11277, #8241, #7216 ) ;
#3471=CIRCLE ( 'NONE', #7416, 4.999999999999976907 ) ;
#3473=ORIENTED_EDGE ( 'NONE', *, *, #12175, .F. ) ;
#3474=DIRECTION ( 'NONE',  ( 0.000000000000000000, 0.000000000000000000, 1.000000000000000000 ) ) ;
#3486=DIRECTION ( 'NONE',  ( 6.608470384673545847E-17, -1.000000000000000000, 0.000000000000000000 ) ) ;
#3493=DIRECTION ( 'NONE',  ( -1.000000000000000000, -1.913084959030911013E-15, -0.000000000000000000 ) ) ;
#3500=CARTESIAN_POINT ( 'NONE',  ( 24.99999999999998934, 189.5765550933606107, -2.000000000000001776 ) ) ;
#3501=ORIENTED_EDGE ( 'NONE', *, *, #4235, .T. ) ;
#3502=CARTESIAN_POINT ( 'NONE',  ( 68.68170757442801744, -83.66032599071898801, -106.9999999999999858 ) ) ;
#3507=CARTESIAN_POINT ( 'NONE',  ( -108.6817075744280316, -30.42344490663958112, -32.00000000000002842 ) ) ;
#3521=ORIENTED_EDGE ( 'NONE', *, *, #9684, .T. ) ;
#3522=AXIS2_PLACEMENT_3D ( 'NONE', #10871, #5091, #6403 ) ;
#3523=DIRECTION ( 'NONE',  ( 0.000000000000000000, 0.000000000000000000, -1.000000000000000000 ) ) ;
#3525=EDGE_CURVE ( 'NONE', #6549, #7848, #2872, .T. ) ;
#3546=FACE_OUTER_BOUND ( 'NONE', #1076, .T. ) ;
#3566=CARTESIAN_POINT ( 'NONE',  ( 68.68170757442801744, 39.57655509336063915, 33.00000000000002842 ) ) ;
#3567=ORIENTED_EDGE ( 'NONE', *, *, #10690, .T. ) ;
#3568=DIRECTION ( 'NONE',  ( -0.000000000000000000, 1.000000000000000000, -0.000000000000000000 ) ) ;
#3569=AXIS2_PLACEMENT_3D ( 'NONE', #7986, #10479, #4841 ) ;
#3577=CIRCLE ( 'NONE', #4514, 4.999999999999988454 ) ;
#3585=DIRECTION ( 'NONE',  ( 0.000000000000000000, 1.000000000000000000, 0.000000000000000000 ) ) ;
#3592=VERTEX_POINT ( 'NONE', #644 ) ;
#3596=CARTESIAN_POINT ( 'NONE',  ( 88.22284556172391490, 29.57655509336062849, -106.9999999999999858 ) ) ;
#3602=DIRECTION ( 'NONE',  ( 0.000000000000000000, 0.000000000000000000, 1.000000000000000000 ) ) ;
#3609=CARTESIAN_POINT ( 'NONE',  ( 129.3408537872138595, 189.5765550933606107, -4.000000000000019540 ) ) ;
#3612=DIRECTION ( 'NONE',  ( -1.000000000000000000, 1.892425610156516875E-16, 0.000000000000000000 ) ) ;
#3616=DIRECTION ( 'NONE',  ( -0.000000000000000000, 1.000000000000000000, -0.000000000000000000 ) ) ;
#3621=EDGE_CURVE ( 'NONE', #7201, #7974, #3415, .T. ) ;
#3625=VERTEX_POINT ( 'NONE', #12185 ) ;
#3626=CYLINDRICAL_SURFACE ( 'NONE', #237, 3.299999999999976730 ) ;
#3640=VERTEX_POINT ( 'NONE', #14457 ) ;
#3645=ORIENTED_EDGE ( 'NONE', *, *, #12264, .F. ) ;
#3654=LINE ( 'NONE', #2619, #9149 ) ;
#3665=LINE ( 'NONE', #5903, #12422 ) ;
#3674=ORIENTED_EDGE ( 'NONE', *, *, #8055, .F. ) ;
#3677=VECTOR ( 'NONE', #1474, 1000.000000000000000 ) ;
#3678=ORIENTED_EDGE ( 'NONE', *, *, #7571, .F. ) ;
#3679=ORIENTED_EDGE ( 'NONE', *, *, #10443, .T. ) ;
#3683=VERTEX_POINT ( 'NONE', #5713 ) ;
#3690=VECTOR ( 'NONE', #3143, 1000.000000000000000 ) ;
#3697=VERTEX_POINT ( 'NONE', #11149 ) ;
#3719=FACE_BOUND ( 'NONE', #1538, .T. ) ;
#3724=EDGE_CURVE ( 'NONE', #6531, #2687, #7850, .T. ) ;
#3737=DIRECTION ( 'NONE',  ( -1.000000000000000000, -1.723842398015259277E-15, 0.000000000000000000 ) ) ;
#3752=DIRECTION ( 'NONE',  ( 0.000000000000000000, 0.000000000000000000, 1.000000000000000000 ) ) ;
#3754=PLANE ( 'NONE',  #11733 ) ;
#3759=CARTESIAN_POINT ( 'NONE',  ( -25.00000000000000000, -30.42444490663959300, 47.99999999999998579 ) ) ;
#3762=DIRECTION ( 'NONE',  ( 0.000000000000000000, 0.000000000000000000, -1.000000000000000000 ) ) ;
#3772=ORIENTED_EDGE ( 'NONE', *, *, #14001, .F. ) ;
#3778=AXIS2_PLACEMENT_3D ( 'NONE', #4822, #3737, #2560 ) ;
#3779=CARTESIAN_POINT ( 'NONE',  ( -140.0000000000003411, 199.5765550933606107, 47.99999999999998579 ) ) ;
#3780=ORIENTED_EDGE ( 'NONE', *, *, #11568, .T. ) ;
#3796=CIRCLE ( 'NONE', #8691, 3.299999999999983391 ) ;
#3799=LINE ( 'NONE', #3507, #1396 ) ;
#3808=ORIENTED_EDGE ( 'NONE', *, *, #14296, .T. ) ;
#3810=ORIENTED_EDGE ( 'NONE', *, *, #10855, .T. ) ;
#3816=ORIENTED_EDGE ( 'NONE', *, *, #3213, .T. ) ;
#3819=FACE_OUTER_BOUND ( 'NONE', #6811, .T. ) ;
#3821=DIRECTION ( 'NONE',  ( 0.000000000000000000, 0.000000000000000000, 1.000000000000000000 ) ) ;
#3843=EDGE_CURVE ( 'NONE', #254, #13727, #10343, .T. ) ;
#3849=( NAMED_UNIT ( * ) SI_UNIT ( $, .STERADIAN. ) SOLID_ANGLE_UNIT ( ) );
#3852=EDGE_CURVE ( 'NONE', #8822, #408, #5666, .T. ) ;
#3867=CARTESIAN_POINT ( 'NONE',  ( -129.3408537872145132, 199.5765550933606107, -80.00000000000001421 ) ) ;
#3870=CARTESIAN_POINT ( 'NONE',  ( 118.6817075744280174, -20.42344490663938927, -117.0000000000000000 ) ) ;
#3874=EDGE_CURVE ( 'NONE', #12513, #2459, #11577, .T. ) ;
#3884=DIRECTION ( 'NONE',  ( 0.000000000000000000, 1.000000000000000000, 0.000000000000000000 ) ) ;
#3892=ORIENTED_EDGE ( 'NONE', *, *, #13707, .T. ) ;
#3893=VERTEX_POINT ( 'NONE', #13935 ) ;
#3917=VERTEX_POINT ( 'NONE', #4140 ) ;
#3920=VERTEX_POINT ( 'NONE', #3042 ) ;
#3928=AXIS2_PLACEMENT_3D ( 'NONE', #9908, #3474, #9305 ) ;
#3933=PLANE ( 'NONE',  #12255 ) ;
#3940=DIRECTION ( 'NONE',  ( 1.913084959030911013E-15, -1.000000000000000000, 0.000000000000000000 ) ) ;
#3943=DIRECTION ( 'NONE',  ( -1.000000000000000000, 0.000000000000000000, -0.000000000000000000 ) ) ;
#3951=PLANE ( 'NONE',  #4993 ) ;
#3953=ORIENTED_EDGE ( 'NONE', *, *, #7524, .T. ) ;
#3957=LINE ( 'NONE', #2864, #3047 ) ;
#3960=CARTESIAN_POINT ( 'NONE',  ( 0.000000000000000000, -30.42444490663959300, -32.00000000000002842 ) ) ;
#3973=ORIENTED_EDGE ( 'NONE', *, *, #2716, .T. ) ;
#3976=ORIENTED_EDGE ( 'NONE', *, *, #6320, .F. ) ;
#3979=ORIENTED_EDGE ( 'NONE', *, *, #11946, .F. ) ;
#3993=PLANE ( 'NONE',  #12653 ) ;
#4004=AXIS2_PLACEMENT_3D ( 'NONE', #11254, #4810, #12558 ) ;
#4034=EDGE_CURVE ( 'NONE', #12216, #7928, #13704, .T. ) ;
#4035=LINE ( 'NONE', #439, #8633 ) ;
#4052=ADVANCED_FACE ( 'NONE', ( #2896 ), #6307, .F. ) ;
#4059=EDGE_CURVE ( 'NONE', #7201, #11896, #10110, .T. ) ;
#4064=EDGE_CURVE ( 'NONE', #2782, #663, #9970, .T. ) ;
#4072=DIRECTION ( 'NONE',  ( 0.000000000000000000, 0.000000000000000000, 1.000000000000000000 ) ) ;
#4077=FACE_BOUND ( 'NONE', #12479, .T. ) ;
#4087=ORIENTED_EDGE ( 'NONE', *, *, #2573, .T. ) ;
#4094=ORIENTED_EDGE ( 'NONE', *, *, #1185, .T. ) ;
#4102=DIRECTION ( 'NONE',  ( 0.000000000000000000, 0.000000000000000000, -1.000000000000000000 ) ) ;
#4115=CYLINDRICAL_SURFACE ( 'NONE', #2813, 4.999999999999988454 ) ;
#4124=ADVANCED_FACE ( 'NONE', ( #3464 ), #3400, .F. ) ;
#4134=AXIS2_PLACEMENT_3D ( 'NONE', #10706, #888, #4072 ) ;
#4140=CARTESIAN_POINT ( 'NONE',  ( 24.99999999999999289, 199.5765550933606107, -2.000000000000001776 ) ) ;
#4141=LINE ( 'NONE', #1933, #3206 ) ;
#4155=DIRECTION ( 'NONE',  ( 0.000000000000000000, 0.000000000000000000, -1.000000000000000000 ) ) ;
#4165=EDGE_CURVE ( 'NONE', #2504, #10603, #8093, .T. ) ;
#4172=AXIS2_PLACEMENT_3D ( 'NONE', #12610, #8221, #5945 ) ;
#4177=DIRECTION ( 'NONE',  ( 0.000000000000000000, 0.000000000000000000, -1.000000000000000000 ) ) ;
#4184=SHAPE_DEFINITION_REPRESENTATION ( #2507, #11805 ) ;
#4218=VERTEX_POINT ( 'NONE', #11413 ) ;
#4225=CARTESIAN_POINT ( 'NONE',  ( 68.68170757442801744, 29.57655509336062849, -106.9999999999999858 ) ) ;
#4235=EDGE_CURVE ( 'NONE', #13862, #6531, #12583, .T. ) ;
#4237=CYLINDRICAL_SURFACE ( 'NONE', #6021, 3.299999999999976730 ) ;
#4239=ORIENTED_EDGE ( 'NONE', *, *, #225, .F. ) ;
#4255=EDGE_CURVE ( 'NONE', #5614, #1477, #4700, .T. ) ;
#4256=CARTESIAN_POINT ( 'NONE',  ( 118.6817075744280316, 109.5765550933604828, -3.299999999999983391 ) ) ;
#4261=PRODUCT_CONTEXT ( 'NONE', #11289, 'mechanical' ) ;
#4267=ADVANCED_FACE ( 'NONE', ( #6883 ), #10177, .T. ) ;
#4279=AXIS2_PLACEMENT_3D ( 'NONE', #570, #8153, #491 ) ;
#4282=AXIS2_PLACEMENT_3D ( 'NONE', #5860, #10347, #4790 ) ;
#4283=DIRECTION ( 'NONE',  ( 0.000000000000000000, -1.000000000000000000, 0.000000000000000000 ) ) ;
#4293=DIRECTION ( 'NONE',  ( 0.000000000000000000, 1.000000000000000000, 0.000000000000000000 ) ) ;
#4297=DIRECTION ( 'NONE',  ( 0.000000000000000000, 1.000000000000000000, 0.000000000000000000 ) ) ;
#4304=EDGE_CURVE ( 'NONE', #1320, #6031, #1697, .T. ) ;
#4307=PLANE ( 'NONE',  #9910 ) ;
#4347=FACE_BOUND ( 'NONE', #935, .T. ) ;
#4349=EDGE_LOOP ( 'NONE', ( #13755, #1986 ) ) ;
#4358=LINE ( 'NONE', #12877, #454 ) ;
#4359=FACE_BOUND ( 'NONE', #1330, .T. ) ;
#4364=CARTESIAN_POINT ( 'NONE',  ( -129.3408537872145132, 189.5765550933606107, -80.00000000000001421 ) ) ;
#4370=EDGE_CURVE ( 'NONE', #768, #12696, #9669, .T. ) ;
#4378=FACE_OUTER_BOUND ( 'NONE', #6790, .T. ) ;
#4418=CARTESIAN_POINT ( 'NONE',  ( 129.3408537872138595, 189.5765550933606107, -75.00000000000001421 ) ) ;
#4446=ORIENTED_EDGE ( 'NONE', *, *, #7029, .F. ) ;
#4476=DIRECTION ( 'NONE',  ( 0.000000000000000000, -1.000000000000000000, 0.000000000000000000 ) ) ;
#4487=DIRECTION ( 'NONE',  ( 0.000000000000000000, 0.000000000000000000, 1.000000000000000000 ) ) ;
#4495=AXIS2_PLACEMENT_3D ( 'NONE', #9513, #2792, #5112 ) ;
#4500=DIRECTION ( 'NONE',  ( 0.000000000000000000, 1.000000000000000000, 0.000000000000000000 ) ) ;
#4504=CARTESIAN_POINT ( 'NONE',  ( -68.68170757442807428, 29.57655509336051125, -117.0000000000000000 ) ) ;
#4506=AXIS2_PLACEMENT_3D ( 'NONE', #12154, #6580, #3523 ) ;
#4509=EDGE_LOOP ( 'NONE', ( #6830, #2649, #794, #11026 ) ) ;
#4511=EDGE_LOOP ( 'NONE', ( #14276, #1496, #13998, #11944 ) ) ;
#4514=AXIS2_PLACEMENT_3D ( 'NONE', #7450, #9445, #807 ) ;
#4556=DIRECTION ( 'NONE',  ( -1.000000000000000000, -1.913084959030911013E-15, -0.000000000000000000 ) ) ;
#4578=VERTEX_POINT ( 'NONE', #12298 ) ;
#4582=CARTESIAN_POINT ( 'NONE',  ( 108.6817075744280743, -20.42344490663954204, -106.9999999999999858 ) ) ;
#4587=LINE ( 'NONE', #13510, #8999 ) ;
#4620=ORIENTED_EDGE ( 'NONE', *, *, #3213, .F. ) ;
#4624=DIRECTION ( 'NONE',  ( 0.000000000000000000, 0.000000000000000000, -1.000000000000000000 ) ) ;
#4638=VECTOR ( 'NONE', #5311, 1000.000000000000000 ) ;
#4649=DIRECTION ( 'NONE',  ( 1.000000000000000000, -0.000000000000000000, -0.000000000000000000 ) ) ;
#4656=DIRECTION ( 'NONE',  ( 0.000000000000000000, -1.000000000000000000, 0.000000000000000000 ) ) ;
#4678=VECTOR ( 'NONE', #10003, 1000.000000000000000 ) ;
#4696=VECTOR ( 'NONE', #1747, 1000.000000000000000 ) ;
#4699=VECTOR ( 'NONE', #6233, 1000.000000000000000 ) ;
#4700=LINE ( 'NONE', #7092, #5532 ) ;
#4703=ORIENTED_EDGE ( 'NONE', *, *, #5569, .T. ) ;
#4711=VERTEX_POINT ( 'NONE', #12439 ) ;
#4727=EDGE_CURVE ( 'NONE', #11896, #663, #149, .T. ) ;
#4730=CARTESIAN_POINT ( 'NONE',  ( 129.3408537872138595, 199.5765550933606107, -9.000000000000007105 ) ) ;
#4742=CARTESIAN_POINT ( 'NONE',  ( 118.6817075744280316, 69.57655509336046862, -3.299999999999983391 ) ) ;
#4749=VECTOR ( 'NONE', #3261, 1000.000000000000000 ) ;
#4756=FACE_OUTER_BOUND ( 'NONE', #10146, .T. ) ;
#4766=ORIENTED_EDGE ( 'NONE', *, *, #10539, .T. ) ;
#4775=ADVANCED_FACE ( 'NONE', ( #3199 ), #12723, .T. ) ;
#4790=DIRECTION ( 'NONE',  ( 0.000000000000000000, 0.000000000000000000, -1.000000000000000000 ) ) ;
#4802=LINE ( 'NONE', #12113, #9681 ) ;
#4808=CARTESIAN_POINT ( 'NONE',  ( -108.6817075744279748, -20.42344490663957046, 33.00000000000002842 ) ) ;
#4810=DIRECTION ( 'NONE',  ( 0.000000000000000000, 0.000000000000000000, 1.000000000000000000 ) ) ;
#4822=CARTESIAN_POINT ( 'NONE',  ( -118.6817075744281595, 69.57655509336025546, 0.000000000000000000 ) ) ;
#4823=CARTESIAN_POINT ( 'NONE',  ( -25.00000000000000000, 199.5765550933606107, 47.99999999999998579 ) ) ;
#4826=DIRECTION ( 'NONE',  ( -1.913084959030911013E-15, 1.000000000000000000, 0.000000000000000000 ) ) ;
#4841=DIRECTION ( 'NONE',  ( -1.892425610156517368E-16, -1.000000000000000000, 0.000000000000000000 ) ) ;
#4846=UNCERTAINTY_MEASURE_WITH_UNIT (LENGTH_MEASURE( 1.000000000000000082E-05 ), #6032, 'distance_accuracy_value', 'NONE');
#4850=CIRCLE ( 'NONE', #1116, 3.299999999999969624 ) ;
#4851=AXIS2_PLACEMENT_3D ( 'NONE', #10890, #6483, #10959 ) ;
#4852=FACE_OUTER_BOUND ( 'NONE', #3049, .T. ) ;
#4857=ORIENTED_EDGE ( 'NONE', *, *, #6320, .T. ) ;
#4863=AXIS2_PLACEMENT_3D ( 'NONE', #8120, #6824, #5705 ) ;
#4878=VECTOR ( 'NONE', #2467, 1000.000000000000000 ) ;
#4887=LINE ( 'NONE', #505, #9672 ) ;
#4893=LINE ( 'NONE', #2634, #13314 ) ;
#4899=AXIS2_PLACEMENT_3D ( 'NONE', #13981, #3884, #5703 ) ;
#4907=AXIS2_PLACEMENT_3D ( 'NONE', #7338, #5360, #1790 ) ;
#4912=EDGE_LOOP ( 'NONE', ( #1695, #9906, #9590, #6566 ) ) ;
#4942=VECTOR ( 'NONE', #4624, 1000.000000000000000 ) ;
#4946=FACE_OUTER_BOUND ( 'NONE', #6715, .T. ) ;
#4964=CARTESIAN_POINT ( 'NONE',  ( 139.9999999999996874, 189.5765550933606107, 47.99999999999998579 ) ) ;
#4965=ORIENTED_EDGE ( 'NONE', *, *, #5036, .F. ) ;
#4966=VERTEX_POINT ( 'NONE', #13582 ) ;
#4968=CARTESIAN_POINT ( 'NONE',  ( -88.22284556172398595, 39.57655509336048283, -117.0000000000000000 ) ) ;
#4975=DIRECTION ( 'NONE',  ( -1.000000000000000000, 0.000000000000000000, -0.000000000000000000 ) ) ;
#4987=DIRECTION ( 'NONE',  ( 0.000000000000000000, 1.000000000000000000, 0.000000000000000000 ) ) ;
#4993=AXIS2_PLACEMENT_3D ( 'NONE', #4964, #11777, #12634 ) ;
#5003=UNCERTAINTY_MEASURE_WITH_UNIT (LENGTH_MEASURE( 1.000000000000000082E-05 ), #13584, 'distance_accuracy_value', 'NONE');
#5008=ORIENTED_EDGE ( 'NONE', *, *, #13645, .T. ) ;
#5011=ORIENTED_EDGE ( 'NONE', *, *, #14287, .F. ) ;
#5014=VERTEX_POINT ( 'NONE', #11224 ) ;
#5023=CARTESIAN_POINT ( 'NONE',  ( 108.6817075744280743, 29.57655509336062849, -106.9999999999999858 ) ) ;
#5035=DIRECTION ( 'NONE',  ( -0.000000000000000000, 1.000000000000000000, -0.000000000000000000 ) ) ;
#5036=EDGE_CURVE ( 'NONE', #2687, #2858, #4587, .T. ) ;
#5040=VERTEX_POINT ( 'NONE', #7925 ) ;
#5045=CARTESIAN_POINT ( 'NONE',  ( -118.6817075744279606, -30.42344490663958112, -117.0000000000000000 ) ) ;
#5047=LINE ( 'NONE', #9355, #7258 ) ;
#5054=VERTEX_POINT ( 'NONE', #470 ) ;
#5060=VECTOR ( 'NONE', #1047, 1000.000000000000000 ) ;
#5078=EDGE_LOOP ( 'NONE', ( #1823, #2960, #13006, #5011 ) ) ;
#5091=DIRECTION ( 'NONE',  ( 1.000000000000000000, 1.723842398015259277E-15, -0.000000000000000000 ) ) ;
#5096=VECTOR ( 'NONE', #6587, 1000.000000000000000 ) ;
#5103=CYLINDRICAL_SURFACE ( 'NONE', #11069, 5.000000000000004441 ) ;
#5107=CIRCLE ( 'NONE', #9558, 3.299999999999983391 ) ;
#5112=DIRECTION ( 'NONE',  ( -1.000000000000000000, 0.000000000000000000, 1.276920294826117846E-16 ) ) ;
#5129=ADVANCED_FACE ( 'NONE', ( #12754, #2741, #13662, #12679, #7183, #11657 ), #7036, .F. ) ;
#5139=VECTOR ( 'NONE', #4293, 1000.000000000000000 ) ;
#5147=FACE_BOUND ( 'NONE', #8613, .T. ) ;
#5162=ORIENTED_EDGE ( 'NONE', *, *, #1139, .F. ) ;
#5177=DIRECTION ( 'NONE',  ( 0.000000000000000000, 1.000000000000000000, -0.000000000000000000 ) ) ;
#5178=VECTOR ( 'NONE', #1759, 1000.000000000000000 ) ;
#5211=ORIENTED_EDGE ( 'NONE', *, *, #6206, .F. ) ;
#5214=AXIS2_PLACEMENT_3D ( 'NONE', #12240, #4500, #13267 ) ;
#5216=EDGE_CURVE ( 'NONE', #10014, #11757, #767, .T. ) ;
#5229=CARTESIAN_POINT ( 'NONE',  ( 6.123233995736776143E-16, 189.5765550933606107, -42.00000000000003553 ) ) ;
#5230=EDGE_LOOP ( 'NONE', ( #2182, #1447, #10425, #8154, #10660, #3810, #9125, #13761 ) ) ;
#5232=VECTOR ( 'NONE', #795, 1000.000000000000000 ) ;
#5241=EDGE_LOOP ( 'NONE', ( #12269, #12765, #9527, #10378 ) ) ;
#5251=DIRECTION ( 'NONE',  ( 0.000000000000000000, 0.000000000000000000, -1.000000000000000000 ) ) ;
#5255=EDGE_CURVE ( 'NONE', #1219, #12216, #7547, .T. ) ;
#5256=ADVANCED_FACE ( 'NONE', ( #2900 ), #2004, .T. ) ;
#5271=ORIENTED_EDGE ( 'NONE', *, *, #10702, .T. ) ;
#5272=ADVANCED_FACE ( 'NONE', ( #694, #5147, #14096, #4077, #6518, #7691, #4359 ), #13276, .T. ) ;
#5279=VERTEX_POINT ( 'NONE', #9126 ) ;
#5306=ORIENTED_EDGE ( 'NONE', *, *, #4727, .T. ) ;
#5307=AXIS2_PLACEMENT_3D ( 'NONE', #900, #8870, #12177 ) ;
#5311=DIRECTION ( 'NONE',  ( -0.000000000000000000, 1.000000000000000000, -0.000000000000000000 ) ) ;
#5333=DIRECTION ( 'NONE',  ( 0.000000000000000000, 1.000000000000000000, 0.000000000000000000 ) ) ;
#5334=ORIENTED_EDGE ( 'NONE', *, *, #13563, .F. ) ;
#5348=VECTOR ( 'NONE', #13452, 1000.000000000000000 ) ;
#5358=CARTESIAN_POINT ( 'NONE',  ( 118.6817075744280316, 69.57655509336046862, 0.000000000000000000 ) ) ;
#5360=DIRECTION ( 'NONE',  ( 0.000000000000000000, 0.000000000000000000, 1.000000000000000000 ) ) ;
#5364=ORIENTED_EDGE ( 'NONE', *, *, #11014, .F. ) ;
#5366=FACE_OUTER_BOUND ( 'NONE', #5230, .T. ) ;
#5370=FACE_OUTER_BOUND ( 'NONE', #998, .T. ) ;
#5381=ORIENTED_EDGE ( 'NONE', *, *, #12032, .T. ) ;
#5385=DIRECTION ( 'NONE',  ( -0.000000000000000000, 1.000000000000000000, -0.000000000000000000 ) ) ;
#5390=VERTEX_POINT ( 'NONE', #12722 ) ;
#5410=VECTOR ( 'NONE', #14065, 1000.000000000000000 ) ;
#5415=CARTESIAN_POINT ( 'NONE',  ( 108.6817075744280459, 109.5765550933604828, 0.000000000000000000 ) ) ;
#5430=VECTOR ( 'NONE', #4987, 1000.000000000000000 ) ;
#5434=DIRECTION ( 'NONE',  ( -1.000000000000000000, 0.000000000000000000, 0.000000000000000000 ) ) ;
#5435=DIRECTION ( 'NONE',  ( 0.000000000000000000, -1.000000000000000000, 0.000000000000000000 ) ) ;
#5439=LINE ( 'NONE', #4364, #2049 ) ;
#5441=DIRECTION ( 'NONE',  ( 1.000000000000000000, 0.000000000000000000, 0.000000000000000000 ) ) ;
#5465=AXIS2_PLACEMENT_3D ( 'NONE', #6832, #12468, #11298 ) ;
#5477=ORIENTED_EDGE ( 'NONE', *, *, #7163, .T. ) ;
#5478=ADVANCED_FACE ( 'NONE', ( #1824 ), #3150, .F. ) ;
#5480=EDGE_LOOP ( 'NONE', ( #8376, #5381, #2658, #12612 ) ) ;
#5489=CARTESIAN_POINT ( 'NONE',  ( 108.6817075744280174, 29.57655509336062849, 33.00000000000002842 ) ) ;
#5494=CARTESIAN_POINT ( 'NONE',  ( 129.3408537872138595, 199.5765550933606107, -69.99999999999998579 ) ) ;
#5501=CARTESIAN_POINT ( 'NONE',  ( -140.0000000000003411, 189.5765550933606107, -132.0000000000000000 ) ) ;
#5506=CARTESIAN_POINT ( 'NONE',  ( -129.3408537872145132, 189.5765550933606107, -9.000000000000007105 ) ) ;
#5532=VECTOR ( 'NONE', #5988, 1000.000000000000000 ) ;
#5547=VECTOR ( 'NONE', #6391, 1000.000000000000000 ) ;
#5558=ADVANCED_FACE ( 'NONE', ( #14131 ), #4115, .F. ) ;
#5569=EDGE_CURVE ( 'NONE', #10014, #13737, #14408, .T. ) ;
#5580=VECTOR ( 'NONE', #2788, 1000.000000000000000 ) ;
#5590=EDGE_LOOP ( 'NONE', ( #2722, #5742, #12452, #8480 ) ) ;
#5594=CARTESIAN_POINT ( 'NONE',  ( 108.6817075744280316, -30.42344490663958112, -32.00000000000002842 ) ) ;
#5599=DIRECTION ( 'NONE',  ( -8.619211990076296383E-16, 1.000000000000000000, 0.000000000000000000 ) ) ;
#5606=DIRECTION ( 'NONE',  ( 0.000000000000000000, 0.000000000000000000, 1.000000000000000000 ) ) ;
#5614=VERTEX_POINT ( 'NONE', #14337 ) ;
#5624=DIRECTION ( 'NONE',  ( -1.000000000000000000, -1.723842398015259277E-15, 0.000000000000000000 ) ) ;
#5627=CYLINDRICAL_SURFACE ( 'NONE', #2615, 5.000000000000018652 ) ;
#5663=FACE_OUTER_BOUND ( 'NONE', #4511, .T. ) ;
#5666=CIRCLE ( 'NONE', #13875, 5.000000000000004441 ) ;
#5668=AXIS2_PLACEMENT_3D ( 'NONE', #4730, #12540, #10271 ) ;
#5679=CARTESIAN_POINT ( 'NONE',  ( -108.6817075744281595, 69.57655509336026967, -3.299999999999976730 ) ) ;
#5693=FACE_OUTER_BOUND ( 'NONE', #13459, .T. ) ;
#5703=DIRECTION ( 'NONE',  ( 0.000000000000000000, 0.000000000000000000, 1.000000000000000000 ) ) ;
#5705=DIRECTION ( 'NONE',  ( 1.913084959030911013E-15, -1.000000000000000000, 0.000000000000000000 ) ) ;
#5713=CARTESIAN_POINT ( 'NONE',  ( -129.3408537872145132, 189.5765550933606107, -13.99999999999998401 ) ) ;
#5724=CARTESIAN_POINT ( 'NONE',  ( -118.6817075744281595, 69.57655509336025546, 0.000000000000000000 ) ) ;
#5742=ORIENTED_EDGE ( 'NONE', *, *, #5255, .T. ) ;
#5757=CARTESIAN_POINT ( 'NONE',  ( -129.3408537872145132, 189.5765550933606107, -13.99999999999998401 ) ) ;
#5761=DIRECTION ( 'NONE',  ( 1.723842398015259277E-15, -1.000000000000000000, 0.000000000000000000 ) ) ;
#5773=VECTOR ( 'NONE', #13586, 1000.000000000000000 ) ;
#5777=FACE_OUTER_BOUND ( 'NONE', #3316, .T. ) ;
#5778=ORIENTED_EDGE ( 'NONE', *, *, #4034, .F. ) ;
#5791=VECTOR ( 'NONE', #12844, 1000.000000000000000 ) ;
#5800=DIRECTION ( 'NONE',  ( 1.000000000000000000, -0.000000000000000000, -0.000000000000000000 ) ) ;
#5812=DIRECTION ( 'NONE',  ( 1.892425610156516875E-16, 1.000000000000000000, 0.000000000000000000 ) ) ;
#5825=AXIS2_PLACEMENT_3D ( 'NONE', #8954, #13444, #1204 ) ;
#5857=EDGE_LOOP ( 'NONE', ( #3976, #13238, #14079, #11487, #9948, #4620, #10499, #9014, #3521, #11903, #10867, #6840 ) ) ;
#5860=CARTESIAN_POINT ( 'NONE',  ( -118.6817075744282306, 109.5765550933602697, 0.000000000000000000 ) ) ;
#5863=VERTEX_POINT ( 'NONE', #1955 ) ;
#5867=CIRCLE ( 'NONE', #9366, 5.000000000000004441 ) ;
#5871=EDGE_CURVE ( 'NONE', #3920, #3697, #2828, .T. ) ;
#5895=VECTOR ( 'NONE', #2082, 1000.000000000000000 ) ;
#5903=CARTESIAN_POINT ( 'NONE',  ( -118.6817075744282306, 109.5765550933602697, 3.299999999999976730 ) ) ;
#5927=ORIENTED_EDGE ( 'NONE', *, *, #225, .T. ) ;
#5940=DIRECTION ( 'NONE',  ( 0.000000000000000000, 0.000000000000000000, 1.000000000000000000 ) ) ;
#5945=DIRECTION ( 'NONE',  ( 0.000000000000000000, 0.000000000000000000, 1.000000000000000000 ) ) ;
#5950=ORIENTED_EDGE ( 'NONE', *, *, #7239, .T. ) ;
#5957=EDGE_CURVE ( 'NONE', #5614, #1344, #115, .T. ) ;
#5959=EDGE_CURVE ( 'NONE', #10361, #10652, #12332, .T. ) ;
#5961=CARTESIAN_POINT ( 'NONE',  ( 118.6817075744280316, 69.57655509336046862, 3.299999999999976730 ) ) ;
#5963=VECTOR ( 'NONE', #11204, 1000.000000000000000 ) ;
#5985=PRODUCT_DEFINITION_CONTEXT ( 'detailed design', #3001, 'design' ) ;
#5988=DIRECTION ( 'NONE',  ( -1.321694076934709169E-16, 1.000000000000000000, -0.000000000000000000 ) ) ;
#5991=EDGE_CURVE ( 'NONE', #1, #1219, #6537, .T. ) ;
#5996=ORIENTED_EDGE ( 'NONE', *, *, #6864, .T. ) ;
#6003=CARTESIAN_POINT ( 'NONE',  ( 6.118061346828462449E-15, -30.42344490663947809, 33.00000000000002842 ) ) ;
#6015=ORIENTED_EDGE ( 'NONE', *, *, #12197, .F. ) ;
#6021=AXIS2_PLACEMENT_3D ( 'NONE', #12117, #8535, #6538 ) ;
#6031=VERTEX_POINT ( 'NONE', #13509 ) ;
#6032=( LENGTH_UNIT ( ) NAMED_UNIT ( * ) SI_UNIT ( .MILLI., .METRE. ) );
#6051=CARTESIAN_POINT ( 'NONE',  ( 118.6817075744280601, 189.5765550933606107, 33.00000000000002842 ) ) ;
#6056=CARTESIAN_POINT ( 'NONE',  ( -140.0000000000003411, 189.5765550933606107, -132.0000000000000000 ) ) ;
#6061=ORIENTED_EDGE ( 'NONE', *, *, #4304, .F. ) ;
#6080=DIRECTION ( 'NONE',  ( 1.000000000000000000, -0.000000000000000000, -0.000000000000000000 ) ) ;
#6087=ORIENTED_EDGE ( 'NONE', *, *, #999, .F. ) ;
#6091=ADVANCED_FACE ( 'NONE', ( #4852 ), #3626, .F. ) ;
#6104=FACE_OUTER_BOUND ( 'NONE', #11127, .T. ) ;
#6105=EDGE_LOOP ( 'NONE', ( #12089, #6398, #9881, #810 ) ) ;
#6116=FACE_OUTER_BOUND ( 'NONE', #9490, .T. ) ;
#6117=PLANE ( 'NONE',  #3469 ) ;
#6129=DIRECTION ( 'NONE',  ( 0.000000000000000000, 0.000000000000000000, 1.000000000000000000 ) ) ;
#6132=DIRECTION ( 'NONE',  ( -0.000000000000000000, 0.000000000000000000, -1.000000000000000000 ) ) ;
#6136=DIRECTION ( 'NONE',  ( -1.000000000000000000, -1.723842398015259277E-15, 0.000000000000000000 ) ) ;
#6168=DIRECTION ( 'NONE',  ( 0.000000000000000000, 0.000000000000000000, 1.000000000000000000 ) ) ;
#6175=ADVANCED_FACE ( 'NONE', ( #1858 ), #6310, .F. ) ;
#6198=CARTESIAN_POINT ( 'NONE',  ( 118.6817075744280316, 109.5765550933604828, 3.299999999999976730 ) ) ;
#6204=CARTESIAN_POINT ( 'NONE',  ( 0.000000000000000000, -30.42444490663959300, -37.00000000000003553 ) ) ;
#6206=EDGE_CURVE ( 'NONE', #6602, #6812, #13346, .T. ) ;
#6209=LINE ( 'NONE', #6051, #5580 ) ;
#6214=DIRECTION ( 'NONE',  ( 0.000000000000000000, 0.000000000000000000, 1.000000000000000000 ) ) ;
#6233=DIRECTION ( 'NONE',  ( -1.000000000000000000, -1.723842398015259277E-15, 0.000000000000000000 ) ) ;
#6244=LINE ( 'NONE', #13338, #4942 ) ;
#6291=VERTEX_POINT ( 'NONE', #6517 ) ;
#6306=LINE ( 'NONE', #14297, #4699 ) ;
#6307=CYLINDRICAL_SURFACE ( 'NONE', #11116, 5.000000000000018652 ) ;
#6310=CYLINDRICAL_SURFACE ( 'NONE', #11450, 3.299999999999976730 ) ;
#6320=EDGE_CURVE ( 'NONE', #5614, #10014, #14231, .T. ) ;
#6331=ORIENTED_EDGE ( 'NONE', *, *, #3621, .F. ) ;
#6339=VECTOR ( 'NONE', #8037, 1000.000000000000000 ) ;
#6347=CIRCLE ( 'NONE', #12195, 5.000000000000004441 ) ;
#6356=EDGE_CURVE ( 'NONE', #1, #7928, #1115, .T. ) ;
#6363=EDGE_CURVE ( 'NONE', #14451, #3625, #4358, .T. ) ;
#6365=ORIENTED_EDGE ( 'NONE', *, *, #12875, .T. ) ;
#6373=EDGE_CURVE ( 'NONE', #7928, #12216, #14254, .T. ) ;
#6374=VERTEX_POINT ( 'NONE', #5045 ) ;
#6379=CIRCLE ( 'NONE', #5668, 4.999999999999988454 ) ;
#6380=DIRECTION ( 'NONE',  ( -1.000000000000000000, -1.913084959030911013E-15, -0.000000000000000000 ) ) ;
#6391=DIRECTION ( 'NONE',  ( 0.000000000000000000, 1.000000000000000000, 0.000000000000000000 ) ) ;
#6398=ORIENTED_EDGE ( 'NONE', *, *, #8142, .F. ) ;
#6403=DIRECTION ( 'NONE',  ( 0.000000000000000000, 0.000000000000000000, -1.000000000000000000 ) ) ;
#6447=EDGE_LOOP ( 'NONE', ( #13595, #14022 ) ) ;
#6453=CARTESIAN_POINT ( 'NONE',  ( 118.6817075744280601, 189.5765550933606107, -117.0000000000000000 ) ) ;
#6461=VECTOR ( 'NONE', #12041, 1000.000000000000000 ) ;
#6475=ORIENTED_EDGE ( 'NONE', *, *, #8362, .F. ) ;
#6483=DIRECTION ( 'NONE',  ( 0.000000000000000000, 1.000000000000000000, -0.000000000000000000 ) ) ;
#6491=ORIENTED_EDGE ( 'NONE', *, *, #12525, .F. ) ;
#6498=CARTESIAN_POINT ( 'NONE',  ( 108.6817075744280459, 109.5765550933604828, 0.000000000000000000 ) ) ;
#6506=EDGE_LOOP ( 'NONE', ( #8283, #5211 ) ) ;
#6515=DIRECTION ( 'NONE',  ( 0.000000000000000000, 1.000000000000000000, 0.000000000000000000 ) ) ;
#6517=CARTESIAN_POINT ( 'NONE',  ( -129.3408537872145132, 199.5765550933606107, -13.99999999999998401 ) ) ;
#6518=FACE_BOUND ( 'NONE', #7040, .T. ) ;
#6519=VECTOR ( 'NONE', #12795, 1000.000000000000000 ) ;
#6524=DIRECTION ( 'NONE',  ( 0.000000000000000000, 0.000000000000000000, 1.000000000000000000 ) ) ;
#6531=VERTEX_POINT ( 'NONE', #441 ) ;
#6533=DIRECTION ( 'NONE',  ( -1.000000000000000000, 1.892425610156516875E-16, 0.000000000000000000 ) ) ;
#6537=CIRCLE ( 'NONE', #5825, 5.000000000000018652 ) ;
#6538=DIRECTION ( 'NONE',  ( 0.000000000000000000, 0.000000000000000000, -1.000000000000000000 ) ) ;
#6549=VERTEX_POINT ( 'NONE', #4256 ) ;
#6551=ORIENTED_EDGE ( 'NONE', *, *, #5991, .T. ) ;
#6566=ORIENTED_EDGE ( 'NONE', *, *, #7378, .F. ) ;
#6572=ORIENTED_EDGE ( 'NONE', *, *, #5957, .T. ) ;
#6576=EDGE_CURVE ( 'NONE', #3917, #4711, #12968, .T. ) ;
#6580=DIRECTION ( 'NONE',  ( 1.000000000000000000, -0.000000000000000000, -0.000000000000000000 ) ) ;
#6585=VECTOR ( 'NONE', #6136, 1000.000000000000000 ) ;
#6587=DIRECTION ( 'NONE',  ( 0.000000000000000000, 1.000000000000000000, 0.000000000000000000 ) ) ;
#6594=CARTESIAN_POINT ( 'NONE',  ( 0.000000000000000000, 189.5765550933606107, 33.00000000000002842 ) ) ;
#6602=VERTEX_POINT ( 'NONE', #2036 ) ;
#6658=ORIENTED_EDGE ( 'NONE', *, *, #12525, .T. ) ;
#6668=CARTESIAN_POINT ( 'NONE',  ( 129.3408537872138595, 189.5765550933606107, -69.99999999999998579 ) ) ;
#6674=DIRECTION ( 'NONE',  ( -8.619211990076296383E-16, 1.000000000000000000, 0.000000000000000000 ) ) ;
#6705=ORIENTED_EDGE ( 'NONE', *, *, #12218, .T. ) ;
#6715=EDGE_LOOP ( 'NONE', ( #12736, #854, #1416, #9331 ) ) ;
#6716=VECTOR ( 'NONE', #8049, 1000.000000000000000 ) ;
#6731=AXIS2_PLACEMENT_3D ( 'NONE', #14436, #12025, #4283 ) ;
#6742=STYLED_ITEM ( 'NONE', ( #347 ), #6797 ) ;
#6743=DIRECTION ( 'NONE',  ( 0.000000000000000000, 0.000000000000000000, -1.000000000000000000 ) ) ;
#6770=AXIS2_PLACEMENT_3D ( 'NONE', #13030, #3080, #4177 ) ;
#6788=ORIENTED_EDGE ( 'NONE', *, *, #1962, .T. ) ;
#6790=EDGE_LOOP ( 'NONE', ( #10676, #9145, #9254, #9026 ) ) ;
#6797=MANIFOLD_SOLID_BREP ( 'Cut-Extrude4', #2436 ) ;
#6798=VECTOR ( 'NONE', #2429, 1000.000000000000000 ) ;
#6802=FACE_OUTER_BOUND ( 'NONE', #5241, .T. ) ;
#6811=EDGE_LOOP ( 'NONE', ( #2780, #2121, #12059, #2521 ) ) ;
#6812=VERTEX_POINT ( 'NONE', #4742 ) ;
#6821=EDGE_CURVE ( 'NONE', #7189, #3625, #12623, .T. ) ;
#6824=DIRECTION ( 'NONE',  ( 1.000000000000000000, 1.913084959030911013E-15, 0.000000000000000000 ) ) ;
#6830=ORIENTED_EDGE ( 'NONE', *, *, #1282, .T. ) ;
#6832=CARTESIAN_POINT ( 'NONE',  ( -24.99999999999998934, -30.42444490663959300, -2.000000000000001776 ) ) ;
#6840=ORIENTED_EDGE ( 'NONE', *, *, #5569, .F. ) ;
#6858=DIRECTION ( 'NONE',  ( -0.000000000000000000, 1.000000000000000000, -0.000000000000000000 ) ) ;
#6860=CARTESIAN_POINT ( 'NONE',  ( -129.3408537872145132, 189.5765550933606107, -4.000000000000031086 ) ) ;
#6864=EDGE_CURVE ( 'NONE', #13172, #5863, #5107, .T. ) ;
#6883=FACE_OUTER_BOUND ( 'NONE', #2369, .T. ) ;
#6894=FACE_OUTER_BOUND ( 'NONE', #1234, .T. ) ;
#6896=AXIS2_PLACEMENT_3D ( 'NONE', #7688, #2068, #10985 ) ;
#6901=ORIENTED_EDGE ( 'NONE', *, *, #784, .T. ) ;
#6920=DIRECTION ( 'NONE',  ( 1.000000000000000000, -0.000000000000000000, -0.000000000000000000 ) ) ;
#6925=EDGE_CURVE ( 'NONE', #6031, #12237, #14422, .T. ) ;
#6927=LINE ( 'NONE', #2477, #2449 ) ;
#6941=PRODUCT_DEFINITION ( 'UNKNOWN', '', #9435, #5985 ) ;
#6949=ORIENTED_EDGE ( 'NONE', *, *, #11946, .T. ) ;
#6954=PLANE ( 'NONE',  #4863 ) ;
#6968=EDGE_CURVE ( 'NONE', #10480, #1551, #14241, .T. ) ;
#6970=CARTESIAN_POINT ( 'NONE',  ( 6.123233995736773185E-16, -30.42444490663959300, -42.00000000000003553 ) ) ;
#7004=LINE ( 'NONE', #11404, #9610 ) ;
#7021=VECTOR ( 'NONE', #12647, 1000.000000000000000 ) ;
#7025=FACE_BOUND ( 'NONE', #6447, .T. ) ;
#7029=EDGE_CURVE ( 'NONE', #13862, #12928, #10140, .T. ) ;
#7036=PLANE ( 'NONE',  #2457 ) ;
#7040=EDGE_LOOP ( 'NONE', ( #6551, #12347 ) ) ;
#7041=DIRECTION ( 'NONE',  ( 1.000000000000000000, 0.000000000000000000, -0.000000000000000000 ) ) ;
#7053=EDGE_LOOP ( 'NONE', ( #8519, #9156, #13557, #8225, #9029, #8892, #737, #5008 ) ) ;
#7054=CARTESIAN_POINT ( 'NONE',  ( -68.68170757442807428, 29.57655509336050415, -106.9999999999999858 ) ) ;
#7066=LINE ( 'NONE', #11685, #8590 ) ;
#7068=VECTOR ( 'NONE', #2891, 1000.000000000000000 ) ;
#7072=EDGE_CURVE ( 'NONE', #10603, #2504, #10240, .T. ) ;
#7090=ORIENTED_EDGE ( 'NONE', *, *, #2464, .T. ) ;
#7092=CARTESIAN_POINT ( 'NONE',  ( 108.6817075744280459, 189.5765550933606107, -106.9999999999999858 ) ) ;
#7100=DIRECTION ( 'NONE',  ( 0.000000000000000000, 0.000000000000000000, 1.000000000000000000 ) ) ;
#7103=EDGE_CURVE ( 'NONE', #4966, #1320, #2310, .T. ) ;
#7104=ORIENTED_EDGE ( 'NONE', *, *, #12875, .F. ) ;
#7105=DIRECTION ( 'NONE',  ( -0.000000000000000000, 1.000000000000000000, -0.000000000000000000 ) ) ;
#7124=ORIENTED_EDGE ( 'NONE', *, *, #10976, .F. ) ;
#7131=DIRECTION ( 'NONE',  ( -2.081668171172169499E-16, 0.000000000000000000, 1.000000000000000000 ) ) ;
#7145=CARTESIAN_POINT ( 'NONE',  ( -24.99999999999998934, 189.5765550933606107, -2.000000000000001776 ) ) ;
#7152=CARTESIAN_POINT ( 'NONE',  ( 129.3408537872138595, 199.5765550933606107, -80.00000000000002842 ) ) ;
#7163=EDGE_CURVE ( 'NONE', #11932, #5040, #11517, .T. ) ;
#7167=AXIS2_PLACEMENT_3D ( 'NONE', #2774, #7214, #3943 ) ;
#7183=FACE_BOUND ( 'NONE', #10459, .T. ) ;
#7184=ORIENTED_EDGE ( 'NONE', *, *, #7427, .T. ) ;
#7189=VERTEX_POINT ( 'NONE', #11441 ) ;
#7201=VERTEX_POINT ( 'NONE', #333 ) ;
#7204=DIRECTION ( 'NONE',  ( 0.000000000000000000, 0.000000000000000000, -1.000000000000000000 ) ) ;
#7210=CARTESIAN_POINT ( 'NONE',  ( -24.99999999999999289, 189.5765550933606107, 47.99999999999998579 ) ) ;
#7214=DIRECTION ( 'NONE',  ( 0.000000000000000000, 0.000000000000000000, -1.000000000000000000 ) ) ;
#7216=DIRECTION ( 'NONE',  ( 0.000000000000000000, 0.000000000000000000, 1.000000000000000000 ) ) ;
#7221=ORIENTED_EDGE ( 'NONE', *, *, #6968, .T. ) ;
#7239=EDGE_CURVE ( 'NONE', #1551, #10480, #4850, .T. ) ;
#7244=VECTOR ( 'NONE', #2054, 1000.000000000000000 ) ;
#7258=VECTOR ( 'NONE', #6132, 1000.000000000000000 ) ;
#7279=ORIENTED_EDGE ( 'NONE', *, *, #10501, .F. ) ;
#7287=AXIS2_PLACEMENT_3D ( 'NONE', #1433, #5800, #7204 ) ;
#7301=ORIENTED_EDGE ( 'NONE', *, *, #3852, .T. ) ;
#7306=DIRECTION ( 'NONE',  ( -1.000000000000000000, -1.723842398015259277E-15, 0.000000000000000000 ) ) ;
#7338=CARTESIAN_POINT ( 'NONE',  ( 0.000000000000000000, 0.000000000000000000, 33.00000000000002842 ) ) ;
#7339=ORIENTED_EDGE ( 'NONE', *, *, #4727, .F. ) ;
#7342=DIRECTION ( 'NONE',  ( 0.000000000000000000, -0.000000000000000000, -1.000000000000000000 ) ) ;
#7361=CARTESIAN_POINT ( 'NONE',  ( -25.00000000000000000, 189.5765550933606107, 47.99999999999998579 ) ) ;
#7363=ADVANCED_FACE ( 'NONE', ( #9396 ), #1941, .F. ) ;
#7378=EDGE_CURVE ( 'NONE', #8822, #10603, #2752, .T. ) ;
#7386=ORIENTED_EDGE ( 'NONE', *, *, #9049, .T. ) ;
#7391=EDGE_CURVE ( 'NONE', #1551, #3920, #10650, .T. ) ;
#7408=ORIENTED_EDGE ( 'NONE', *, *, #4370, .F. ) ;
#7416=AXIS2_PLACEMENT_3D ( 'NONE', #10078, #12282, #5606 ) ;
#7427=EDGE_CURVE ( 'NONE', #5863, #13172, #12100, .T. ) ;
#7439=MECHANICAL_DESIGN_GEOMETRIC_PRESENTATION_REPRESENTATION('',(#6742),#11409);
#7440=CARTESIAN_POINT ( 'NONE',  ( 129.3408537872138595, 189.5765550933606107, -9.000000000000007105 ) ) ;
#7450=CARTESIAN_POINT ( 'NONE',  ( 129.3408537872138595, 199.5765550933606107, -9.000000000000007105 ) ) ;
#7494=CARTESIAN_POINT ( 'NONE',  ( 88.22284556172391490, 29.57655509336062849, -117.0000000000000000 ) ) ;
#7524=EDGE_CURVE ( 'NONE', #4218, #13865, #26, .T. ) ;
#7527=ORIENTED_EDGE ( 'NONE', *, *, #5957, .F. ) ;
#7532=AXIS2_PLACEMENT_3D ( 'NONE', #7589, #3612, #4476 ) ;
#7534=EDGE_CURVE ( 'NONE', #408, #2504, #5439, .T. ) ;
#7547=LINE ( 'NONE', #12034, #5139 ) ;
#7549=ADVANCED_FACE ( 'NONE', ( #8801 ), #8732, .T. ) ;
#7557=CARTESIAN_POINT ( 'NONE',  ( -140.0000000000003411, 189.5765550933606107, 47.99999999999998579 ) ) ;
#7561=LINE ( 'NONE', #14318, #10846 ) ;
#7569=ORIENTED_EDGE ( 'NONE', *, *, #37, .T. ) ;
#7571=EDGE_CURVE ( 'NONE', #3393, #3463, #2078, .T. ) ;
#7575=AXIS2_PLACEMENT_3D ( 'NONE', #6498, #3226, #10835 ) ;
#7589=CARTESIAN_POINT ( 'NONE',  ( 108.6817075744280316, 69.57655509336046862, 0.000000000000000000 ) ) ;
#7592=ORIENTED_EDGE ( 'NONE', *, *, #9187, .F. ) ;
#7603=ADVANCED_FACE ( 'NONE', ( #5366 ), #10994, .T. ) ;
#7608=LINE ( 'NONE', #887, #7953 ) ;
#7622=ADVANCED_FACE ( 'NONE', ( #3546 ), #9154, .F. ) ;
#7623=ORIENTED_EDGE ( 'NONE', *, *, #13681, .F. ) ;
#7626=CARTESIAN_POINT ( 'NONE',  ( 108.6817075744280174, -30.42344490663958112, 47.99999999999998579 ) ) ;
#7638=AXIS2_PLACEMENT_3D ( 'NONE', #9697, #14169, #972 ) ;
#7642=EDGE_CURVE ( 'NONE', #7974, #10568, #11212, .T. ) ;
#7671=DIRECTION ( 'NONE',  ( 0.000000000000000000, 0.000000000000000000, 1.000000000000000000 ) ) ;
#7688=CARTESIAN_POINT ( 'NONE',  ( -129.3408537872145132, 199.5765550933606107, -75.00000000000001421 ) ) ;
#7689=LINE ( 'NONE', #4504, #5060 ) ;
#7691=FACE_OUTER_BOUND ( 'NONE', #10255, .T. ) ;
#7704=ADVANCED_FACE ( 'NONE', ( #10333, #7025, #13649 ), #6954, .F. ) ;
#7714=CARTESIAN_POINT ( 'NONE',  ( -108.6817075744279890, 189.5765550933605823, -106.9999999999999858 ) ) ;
#7716=CARTESIAN_POINT ( 'NONE',  ( 68.68170757442801744, 29.57655509336062849, 33.00000000000002842 ) ) ;
#7723=EDGE_LOOP ( 'NONE', ( #7221, #5950 ) ) ;
#7724=AXIS2_PLACEMENT_3D ( 'NONE', #13205, #6380, #1785 ) ;
#7744=AXIS2_PLACEMENT_3D ( 'NONE', #2699, #11464, #8024 ) ;
#7748=ORIENTED_EDGE ( 'NONE', *, *, #11297, .F. ) ;
#7751=CARTESIAN_POINT ( 'NONE',  ( -129.3408537872145132, 199.5765550933606107, -4.000000000000031086 ) ) ;
#7753=CYLINDRICAL_SURFACE ( 'NONE', #4506, 3.299999999999976730 ) ;
#7758=VERTEX_POINT ( 'NONE', #12825 ) ;
#7783=LINE ( 'NONE', #11219, #14361 ) ;
#7807=EDGE_LOOP ( 'NONE', ( #12734, #105, #13490, #10440 ) ) ;
#7837=CARTESIAN_POINT ( 'NONE',  ( 129.3408537872138595, 189.5765550933606107, -9.000000000000007105 ) ) ;
#7848=VERTEX_POINT ( 'NONE', #11128 ) ;
#7850=LINE ( 'NONE', #11086, #9863 ) ;
#7854=SURFACE_STYLE_USAGE ( .BOTH. , #11303 ) ;
#7868=VECTOR ( 'NONE', #7131, 1000.000000000000000 ) ;
#7881=EDGE_CURVE ( 'NONE', #5390, #12237, #8715, .T. ) ;
#7908=ORIENTED_EDGE ( 'NONE', *, *, #6373, .F. ) ;
#7925=CARTESIAN_POINT ( 'NONE',  ( 6.123233995736776143E-16, 199.5765550933606107, -42.00000000000003553 ) ) ;
#7928=VERTEX_POINT ( 'NONE', #5494 ) ;
#7952=VECTOR ( 'NONE', #5434, 1000.000000000000000 ) ;
#7953=VECTOR ( 'NONE', #14372, 1000.000000000000000 ) ;
#7962=CYLINDRICAL_SURFACE ( 'NONE', #3778, 3.299999999999976730 ) ;
#7972=VECTOR ( 'NONE', #300, 1000.000000000000000 ) ;
#7974=VERTEX_POINT ( 'NONE', #3241 ) ;
#7975=ORIENTED_EDGE ( 'NONE', *, *, #1185, .F. ) ;
#7986=CARTESIAN_POINT ( 'NONE',  ( 118.6817075744280174, -20.42344490663938927, 33.00000000000002842 ) ) ;
#7993=EDGE_CURVE ( 'NONE', #433, #3592, #9053, .T. ) ;
#7999=ORIENTED_EDGE ( 'NONE', *, *, #1579, .T. ) ;
#8007=AXIS2_PLACEMENT_3D ( 'NONE', #8053, #463, #539 ) ;
#8008=EDGE_LOOP ( 'NONE', ( #9476, #13576, #3355, #14212 ) ) ;
#8024=DIRECTION ( 'NONE',  ( 0.000000000000000000, 0.000000000000000000, 1.000000000000000000 ) ) ;
#8037=DIRECTION ( 'NONE',  ( 1.000000000000000000, 0.000000000000000000, -0.000000000000000000 ) ) ;
#8044=ADVANCED_FACE ( 'NONE', ( #10376 ), #6117, .T. ) ;
#8049=DIRECTION ( 'NONE',  ( -1.000000000000000000, -0.000000000000000000, 1.276920294826117846E-16 ) ) ;
#8053=CARTESIAN_POINT ( 'NONE',  ( -118.6817075744281595, 69.57655509336025546, 0.000000000000000000 ) ) ;
#8055=EDGE_CURVE ( 'NONE', #562, #3917, #7066, .T. ) ;
#8077=PLANE ( 'NONE',  #10138 ) ;
#8078=PLANE ( 'NONE',  #4279 ) ;
#8093=CIRCLE ( 'NONE', #6896, 5.000000000000004441 ) ;
#8110=VECTOR ( 'NONE', #8660, 1000.000000000000000 ) ;
#8120=CARTESIAN_POINT ( 'NONE',  ( -118.6817075744279748, -20.42344490663959178, 33.00000000000002842 ) ) ;
#8137=CYLINDRICAL_SURFACE ( 'NONE', #4282, 3.299999999999976730 ) ;
#8139=PLANE ( 'NONE',  #1668 ) ;
#8142=EDGE_CURVE ( 'NONE', #10034, #11932, #10473, .T. ) ;
#8150=ORIENTED_EDGE ( 'NONE', *, *, #7391, .F. ) ;
#8153=DIRECTION ( 'NONE',  ( -1.000000000000000000, 0.000000000000000000, -2.081668171172169499E-16 ) ) ;
#8154=ORIENTED_EDGE ( 'NONE', *, *, #13134, .F. ) ;
#8158=FILL_AREA_STYLE ('',( #275 ) ) ;
#8160=FACE_BOUND ( 'NONE', #7723, .T. ) ;
#8164=DIRECTION ( 'NONE',  ( -2.081668171172168760E-16, 0.000000000000000000, -1.000000000000000000 ) ) ;
#8191=ORIENTED_EDGE ( 'NONE', *, *, #3251, .F. ) ;
#8201=CARTESIAN_POINT ( 'NONE',  ( -108.6817075744280316, -30.42344490663958112, -32.00000000000002842 ) ) ;
#8208=DIRECTION ( 'NONE',  ( 0.000000000000000000, 1.000000000000000000, -0.000000000000000000 ) ) ;
#8221=DIRECTION ( 'NONE',  ( 0.000000000000000000, 1.000000000000000000, 0.000000000000000000 ) ) ;
#8222=DIRECTION ( 'NONE',  ( 1.000000000000000000, 0.000000000000000000, 0.000000000000000000 ) ) ;
#8225=ORIENTED_EDGE ( 'NONE', *, *, #409, .T. ) ;
#8234=( NAMED_UNIT ( * ) PLANE_ANGLE_UNIT ( ) SI_UNIT ( $, .RADIAN. ) );
#8241=DIRECTION ( 'NONE',  ( 1.000000000000000000, 1.723842398015259277E-15, -0.000000000000000000 ) ) ;
#8283=ORIENTED_EDGE ( 'NONE', *, *, #3260, .F. ) ;
#8312=DIRECTION ( 'NONE',  ( 1.734723475976807094E-16, -0.000000000000000000, 1.000000000000000000 ) ) ;
#8318=CARTESIAN_POINT ( 'NONE',  ( -108.6817075744279748, -20.42344490663957046, 33.00000000000002842 ) ) ;
#8326=EDGE_CURVE ( 'NONE', #10731, #3034, #9929, .T. ) ;
#8327=CARTESIAN_POINT ( 'NONE',  ( -140.0000000000003411, 199.5765550933606107, 47.99999999999998579 ) ) ;
#8340=VECTOR ( 'NONE', #12105, 1000.000000000000000 ) ;
#8362=EDGE_CURVE ( 'NONE', #7974, #4218, #12023, .T. ) ;
#8366=CARTESIAN_POINT ( 'NONE',  ( -118.6817075744281595, 69.57655509336025546, 3.299999999999976730 ) ) ;
#8376=ORIENTED_EDGE ( 'NONE', *, *, #12229, .F. ) ;
#8382=ADVANCED_FACE ( 'NONE', ( #5663 ), #10142, .F. ) ;
#8385=CARTESIAN_POINT ( 'NONE',  ( -108.6817075744280316, -30.42344490663957401, -32.00000000000002842 ) ) ;
#8387=FACE_BOUND ( 'NONE', #919, .T. ) ;
#8392=FACE_OUTER_BOUND ( 'NONE', #6105, .T. ) ;
#8405=DIRECTION ( 'NONE',  ( 0.000000000000000000, 1.000000000000000000, 0.000000000000000000 ) ) ;
#8441=CARTESIAN_POINT ( 'NONE',  ( -88.22284556172397174, 29.57655509336047572, -117.0000000000000000 ) ) ;
#8451=CARTESIAN_POINT ( 'NONE',  ( 25.00000000000000000, 199.5765550933606107, 47.99999999999998579 ) ) ;
#8462=ADVANCED_FACE ( 'NONE', ( #9401 ), #11311, .F. ) ;
#8469=CARTESIAN_POINT ( 'NONE',  ( 129.3408537872138595, 189.5765550933606107, -9.000000000000007105 ) ) ;
#8480=ORIENTED_EDGE ( 'NONE', *, *, #6356, .F. ) ;
#8513=ORIENTED_EDGE ( 'NONE', *, *, #10574, .F. ) ;
#8519=ORIENTED_EDGE ( 'NONE', *, *, #11066, .F. ) ;
#8531=CARTESIAN_POINT ( 'NONE',  ( 108.6817075744280174, -20.42344490663938572, 33.00000000000002842 ) ) ;
#8535=DIRECTION ( 'NONE',  ( 1.000000000000000000, -0.000000000000000000, -0.000000000000000000 ) ) ;
#8556=CARTESIAN_POINT ( 'NONE',  ( -88.22284556172397174, 29.57655509336047572, 33.00000000000002842 ) ) ;
#8561=EDGE_LOOP ( 'NONE', ( #13814, #13690, #8885, #10525 ) ) ;
#8570=CARTESIAN_POINT ( 'NONE',  ( 68.68170757442801744, -83.66032599071898801, 33.00000000000002842 ) ) ;
#8577=DIRECTION ( 'NONE',  ( 0.000000000000000000, 0.000000000000000000, -1.000000000000000000 ) ) ;
#8580=CARTESIAN_POINT ( 'NONE',  ( 0.000000000000000000, 189.5765550933606107, -32.00000000000002842 ) ) ;
#8582=EDGE_LOOP ( 'NONE', ( #12881, #6061, #8912, #13388 ) ) ;
#8587=ORIENTED_EDGE ( 'NONE', *, *, #898, .F. ) ;
#8590=VECTOR ( 'NONE', #2350, 1000.000000000000000 ) ;
#8602=FACE_OUTER_BOUND ( 'NONE', #3044, .T. ) ;
#8613=EDGE_LOOP ( 'NONE', ( #9864, #2166 ) ) ;
#8625=CARTESIAN_POINT ( 'NONE',  ( 108.6817075744280174, -20.42344490663938572, 33.00000000000002842 ) ) ;
#8633=VECTOR ( 'NONE', #12966, 1000.000000000000000 ) ;
#8635=EDGE_CURVE ( 'NONE', #10731, #3393, #14310, .T. ) ;
#8660=DIRECTION ( 'NONE',  ( 0.000000000000000000, 1.000000000000000000, 0.000000000000000000 ) ) ;
#8668=AXIS2_PLACEMENT_3D ( 'NONE', #11516, #13666, #5940 ) ;
#8682=CIRCLE ( 'NONE', #10308, 4.999999999999976907 ) ;
#8691=AXIS2_PLACEMENT_3D ( 'NONE', #1324, #236, #9306 ) ;
#8708=VERTEX_POINT ( 'NONE', #6453 ) ;
#8715=LINE ( 'NONE', #13052, #5096 ) ;
#8718=LINE ( 'NONE', #8570, #7068 ) ;
#8732=PLANE ( 'NONE',  #10220 ) ;
#8733=ADVANCED_FACE ( 'NONE', ( #5370 ), #9980, .F. ) ;
#8758=CARTESIAN_POINT ( 'NONE',  ( -129.3408537872145132, 189.5765550933606107, -80.00000000000001421 ) ) ;
#8795=CARTESIAN_POINT ( 'NONE',  ( 0.000000000000000000, 189.5765550933606107, 0.000000000000000000 ) ) ;
#8801=FACE_OUTER_BOUND ( 'NONE', #3073, .T. ) ;
#8810=DIRECTION ( 'NONE',  ( 0.000000000000000000, 0.000000000000000000, -1.000000000000000000 ) ) ;
#8821=AXIS2_PLACEMENT_3D ( 'NONE', #8469, #5177, #5251 ) ;
#8822=VERTEX_POINT ( 'NONE', #1365 ) ;
#8836=CARTESIAN_POINT ( 'NONE',  ( -140.0000000000003411, 189.5765550933606107, 47.99999999999998579 ) ) ;
#8840=ORIENTED_EDGE ( 'NONE', *, *, #13785, .F. ) ;
#8848=CARTESIAN_POINT ( 'NONE',  ( 0.000000000000000000, 199.5765550933606107, -37.00000000000003553 ) ) ;
#8853=EDGE_LOOP ( 'NONE', ( #7623, #3678, #3075, #10575 ) ) ;
#8860=CARTESIAN_POINT ( 'NONE',  ( -108.6817075744280743, 29.57655509336044020, -117.0000000000000000 ) ) ;
#8868=AXIS2_PLACEMENT_3D ( 'NONE', #8795, #5435, #2073 ) ;
#8870=DIRECTION ( 'NONE',  ( 1.000000000000000000, 0.000000000000000000, -2.081668171172168760E-16 ) ) ;
#8871=EDGE_CURVE ( 'NONE', #1934, #9323, #2051, .T. ) ;
#8876=PLANE ( 'NONE',  #10617 ) ;
#8885=ORIENTED_EDGE ( 'NONE', *, *, #7427, .F. ) ;
#8892=ORIENTED_EDGE ( 'NONE', *, *, #13785, .T. ) ;
#8910=ADVANCED_FACE ( 'NONE', ( #847 ), #2931, .F. ) ;
#8912=ORIENTED_EDGE ( 'NONE', *, *, #10296, .T. ) ;
#8954=CARTESIAN_POINT ( 'NONE',  ( 129.3408537872138595, 189.5765550933606107, -75.00000000000001421 ) ) ;
#8999=VECTOR ( 'NONE', #3486, 1000.000000000000000 ) ;
#9014=ORIENTED_EDGE ( 'NONE', *, *, #6363, .T. ) ;
#9015=PLANE ( 'NONE',  #5465 ) ;
#9026=ORIENTED_EDGE ( 'NONE', *, *, #3260, .T. ) ;
#9029=ORIENTED_EDGE ( 'NONE', *, *, #13681, .T. ) ;
#9034=VERTEX_POINT ( 'NONE', #3153 ) ;
#9049=EDGE_CURVE ( 'NONE', #9323, #1934, #13519, .T. ) ;
#9053=CIRCLE ( 'NONE', #6731, 3.299999999999969624 ) ;
#9073=CARTESIAN_POINT ( 'NONE',  ( -129.3408537872145132, 189.5765550933606107, -75.00000000000001421 ) ) ;
#9091=CARTESIAN_POINT ( 'NONE',  ( 118.6817075744280316, 109.5765550933604828, 0.000000000000000000 ) ) ;
#9104=VECTOR ( 'NONE', #14392, 1000.000000000000000 ) ;
#9125=ORIENTED_EDGE ( 'NONE', *, *, #4235, .F. ) ;
#9126=CARTESIAN_POINT ( 'NONE',  ( -108.6817075744280743, 29.57655509336044020, 33.00000000000002842 ) ) ;
#9145=ORIENTED_EDGE ( 'NONE', *, *, #11014, .T. ) ;
#9149=VECTOR ( 'NONE', #5812, 1000.000000000000000 ) ;
#9154=CYLINDRICAL_SURFACE ( 'NONE', #2058, 5.000000000000004441 ) ;
#9156=ORIENTED_EDGE ( 'NONE', *, *, #6576, .F. ) ;
#9158=AXIS2_PLACEMENT_3D ( 'NONE', #9591, #10541, #13041 ) ;
#9170=FACE_OUTER_BOUND ( 'NONE', #11117, .T. ) ;
#9187=EDGE_CURVE ( 'NONE', #10652, #6291, #3471, .T. ) ;
#9193=LINE ( 'NONE', #352, #2124 ) ;
#9230=PLANE ( 'NONE',  #3569 ) ;
#9232=LINE ( 'NONE', #10338, #1956 ) ;
#9241=FILL_AREA_STYLE ('',( #10263 ) ) ;
#9254=ORIENTED_EDGE ( 'NONE', *, *, #130, .T. ) ;
#9256=ORIENTED_EDGE ( 'NONE', *, *, #10690, .F. ) ;
#9289=CARTESIAN_POINT ( 'NONE',  ( 0.000000000000000000, 199.5765550933606107, -32.00000000000002842 ) ) ;
#9302=ORIENTED_EDGE ( 'NONE', *, *, #13450, .T. ) ;
#9305=DIRECTION ( 'NONE',  ( 1.000000000000000000, 0.000000000000000000, -0.000000000000000000 ) ) ;
#9306=DIRECTION ( 'NONE',  ( 0.000000000000000000, 0.000000000000000000, -1.000000000000000000 ) ) ;
#9312=CARTESIAN_POINT ( 'NONE',  ( -88.22284556172398595, 39.57655509336048283, 33.00000000000002842 ) ) ;
#9318=VERTEX_POINT ( 'NONE', #7210 ) ;
#9323=VERTEX_POINT ( 'NONE', #1812 ) ;
#9331=ORIENTED_EDGE ( 'NONE', *, *, #7881, .F. ) ;
#9337=LINE ( 'NONE', #714, #1325 ) ;
#9343=FACE_OUTER_BOUND ( 'NONE', #13915, .T. ) ;
#9355=CARTESIAN_POINT ( 'NONE',  ( -118.6817075744279606, -30.42344490663958112, 33.00000000000002842 ) ) ;
#9362=LINE ( 'NONE', #2795, #10319 ) ;
#9366=AXIS2_PLACEMENT_3D ( 'NONE', #8848, #14285, #4487 ) ;
#9369=AXIS2_PLACEMENT_3D ( 'NONE', #9073, #1319, #380 ) ;
#9389=CARTESIAN_POINT ( 'NONE',  ( 118.6817075744280316, 109.5765550933604828, 0.000000000000000000 ) ) ;
#9396=FACE_OUTER_BOUND ( 'NONE', #4912, .T. ) ;
#9399=DIRECTION ( 'NONE',  ( -1.000000000000000000, -1.723842398015259277E-15, 0.000000000000000000 ) ) ;
#9401=FACE_OUTER_BOUND ( 'NONE', #5078, .T. ) ;
#9409=ADVANCED_FACE ( 'NONE', ( #9494, #3719, #8160 ), #2614, .T. ) ;
#9425=VECTOR ( 'NONE', #2510, 1000.000000000000000 ) ;
#9435=PRODUCT_DEFINITION_FORMATION_WITH_SPECIFIED_SOURCE ( 'ANY', '', #12326, .NOT_KNOWN. ) ;
#9445=DIRECTION ( 'NONE',  ( 0.000000000000000000, 1.000000000000000000, -0.000000000000000000 ) ) ;
#9449=CARTESIAN_POINT ( 'NONE',  ( 108.6817075744280174, 29.57655509336062849, -117.0000000000000000 ) ) ;
#9473=EDGE_CURVE ( 'NONE', #9034, #6549, #1066, .T. ) ;
#9476=ORIENTED_EDGE ( 'NONE', *, *, #8055, .T. ) ;
#9477=CARTESIAN_POINT ( 'NONE',  ( -129.3408537872145132, 189.5765550933606107, -75.00000000000001421 ) ) ;
#9480=VERTEX_POINT ( 'NONE', #7716 ) ;
#9487=ORIENTED_EDGE ( 'NONE', *, *, #1282, .F. ) ;
#9490=EDGE_LOOP ( 'NONE', ( #3382, #6572, #12651, #3473 ) ) ;
#9494=FACE_OUTER_BOUND ( 'NONE', #2478, .T. ) ;
#9499=CARTESIAN_POINT ( 'NONE',  ( 108.6817075744280174, -20.42344490663938572, 33.00000000000002842 ) ) ;
#9501=ORIENTED_EDGE ( 'NONE', *, *, #13563, .T. ) ;
#9513=CARTESIAN_POINT ( 'NONE',  ( -108.6817075744280316, -30.42344490663958112, -32.00000000000002842 ) ) ;
#9524=DIRECTION ( 'NONE',  ( 0.000000000000000000, 0.000000000000000000, 1.000000000000000000 ) ) ;
#9527=ORIENTED_EDGE ( 'NONE', *, *, #6356, .T. ) ;
#9558=AXIS2_PLACEMENT_3D ( 'NONE', #14184, #14046, #4102 ) ;
#9566=LINE ( 'NONE', #7361, #7868 ) ;
#9571=ORIENTED_EDGE ( 'NONE', *, *, #9684, .F. ) ;
#9587=DIRECTION ( 'NONE',  ( 0.000000000000000000, 0.000000000000000000, 1.000000000000000000 ) ) ;
#9590=ORIENTED_EDGE ( 'NONE', *, *, #4165, .T. ) ;
#9591=CARTESIAN_POINT ( 'NONE',  ( -129.3408537872145132, 189.5765550933606107, -9.000000000000007105 ) ) ;
#9602=CARTESIAN_POINT ( 'NONE',  ( -118.6817075744283727, 189.5765550933606107, -117.0000000000000000 ) ) ;
#9610=VECTOR ( 'NONE', #12646, 1000.000000000000000 ) ;
#9612=VECTOR ( 'NONE', #4826, 1000.000000000000000 ) ;
#9647=ORIENTED_EDGE ( 'NONE', *, *, #6363, .F. ) ;
#9659=DIRECTION ( 'NONE',  ( 0.000000000000000000, 1.000000000000000000, 0.000000000000000000 ) ) ;
#9669=LINE ( 'NONE', #9449, #13634 ) ;
#9672=VECTOR ( 'NONE', #8312, 1000.000000000000000 ) ;
#9681=VECTOR ( 'NONE', #3059, 1000.000000000000000 ) ;
#9684=EDGE_CURVE ( 'NONE', #3625, #13865, #252, .T. ) ;
#9697=CARTESIAN_POINT ( 'NONE',  ( -118.6817075744282306, 109.5765550933602697, 0.000000000000000000 ) ) ;
#9703=ORIENTED_EDGE ( 'NONE', *, *, #3251, .T. ) ;
#9714=CARTESIAN_POINT ( 'NONE',  ( 0.000000000000000000, 189.5765550933606107, -37.00000000000003553 ) ) ;
#9765=ORIENTED_EDGE ( 'NONE', *, *, #10470, .F. ) ;
#9796=CARTESIAN_POINT ( 'NONE',  ( -129.3408537872145132, 199.5765550933606107, -9.000000000000007105 ) ) ;
#9802=ORIENTED_EDGE ( 'NONE', *, *, #7103, .T. ) ;
#9828=CARTESIAN_POINT ( 'NONE',  ( 108.6817075744280174, -20.42344490663938572, 33.00000000000002842 ) ) ;
#9833=AXIS2_PLACEMENT_3D ( 'NONE', #4968, #2092, #6129 ) ;
#9837=AXIS2_PLACEMENT_3D ( 'NONE', #14135, #1829, #10451 ) ;
#9838=CIRCLE ( 'NONE', #8668, 4.999999999999976907 ) ;
#9842=ORIENTED_EDGE ( 'NONE', *, *, #3525, .F. ) ;
#9855=VECTOR ( 'NONE', #3602, 1000.000000000000000 ) ;
#9859=ADVANCED_FACE ( 'NONE', ( #14026 ), #3993, .T. ) ;
#9861=ORIENTED_EDGE ( 'NONE', *, *, #5216, .F. ) ;
#9863=VECTOR ( 'NONE', #8810, 1000.000000000000000 ) ;
#9864=ORIENTED_EDGE ( 'NONE', *, *, #11840, .T. ) ;
#9868=ADVANCED_FACE ( 'NONE', ( #11819 ), #8137, .F. ) ;
#9881=ORIENTED_EDGE ( 'NONE', *, *, #10976, .T. ) ;
#9897=DIRECTION ( 'NONE',  ( -2.081668171172169006E-16, 0.000000000000000000, -1.000000000000000000 ) ) ;
#9906=ORIENTED_EDGE ( 'NONE', *, *, #7534, .T. ) ;
#9908=CARTESIAN_POINT ( 'NONE',  ( 0.000000000000000000, 0.000000000000000000, 33.00000000000002842 ) ) ;
#9910=AXIS2_PLACEMENT_3D ( 'NONE', #8531, #6533, #11003 ) ;
#9927=DIRECTION ( 'NONE',  ( -1.913084959030911013E-15, 1.000000000000000000, 0.000000000000000000 ) ) ;
#9929=LINE ( 'NONE', #997, #13269 ) ;
#9932=ORIENTED_EDGE ( 'NONE', *, *, #13707, .F. ) ;
#9948=ORIENTED_EDGE ( 'NONE', *, *, #2177, .F. ) ;
#9970=LINE ( 'NONE', #6594, #1779 ) ;
#9978=EDGE_LOOP ( 'NONE', ( #7184, #5996 ) ) ;
#9980=PLANE ( 'NONE',  #5307 ) ;
#9981=CARTESIAN_POINT ( 'NONE',  ( -118.6817075744283727, 189.5765550933606107, 33.00000000000002842 ) ) ;
#10003=DIRECTION ( 'NONE',  ( 0.000000000000000000, -1.000000000000000000, 0.000000000000000000 ) ) ;
#10014=VERTEX_POINT ( 'NONE', #13146 ) ;
#10017=ORIENTED_EDGE ( 'NONE', *, *, #14296, .F. ) ;
#10023=CARTESIAN_POINT ( 'NONE',  ( 25.00000000000000000, 199.5765550933606107, 47.99999999999998579 ) ) ;
#10034=VERTEX_POINT ( 'NONE', #8580 ) ;
#10040=CARTESIAN_POINT ( 'NONE',  ( 88.22284556172391490, 39.57655509336063915, -106.9999999999999858 ) ) ;
#10044=ORIENTED_EDGE ( 'NONE', *, *, #9473, .T. ) ;
#10048=EDGE_LOOP ( 'NONE', ( #6705, #13129, #12104, #9932 ) ) ;
#10051=ORIENTED_EDGE ( 'NONE', *, *, #2177, .T. ) ;
#10067=VERTEX_POINT ( 'NONE', #9289 ) ;
#10078=CARTESIAN_POINT ( 'NONE',  ( -129.3408537872145132, 199.5765550933606107, -9.000000000000007105 ) ) ;
#10110=LINE ( 'NONE', #14298, #5963 ) ;
#10124=ADVANCED_FACE ( 'NONE', ( #3819 ), #12169, .F. ) ;
#10127=FACE_OUTER_BOUND ( 'NONE', #8008, .T. ) ;
#10138=AXIS2_PLACEMENT_3D ( 'NONE', #3363, #5599, #1432 ) ;
#10140=LINE ( 'NONE', #11232, #5348 ) ;
#10142=CYLINDRICAL_SURFACE ( 'NONE', #4172, 5.000000000000004441 ) ;
#10146=EDGE_LOOP ( 'NONE', ( #8150, #13735, #14347, #10933 ) ) ;
#10160=ORIENTED_EDGE ( 'NONE', *, *, #3346, .F. ) ;
#10166=DIRECTION ( 'NONE',  ( 1.892425610156517122E-16, 1.000000000000000000, 0.000000000000000000 ) ) ;
#10177=PLANE ( 'NONE',  #615 ) ;
#10197=ORIENTED_EDGE ( 'NONE', *, *, #2136, .F. ) ;
#10200=DIRECTION ( 'NONE',  ( -1.000000000000000000, -1.723842398015259277E-15, 0.000000000000000000 ) ) ;
#10201=EDGE_CURVE ( 'NONE', #14013, #5279, #11930, .T. ) ;
#10203=ADVANCED_FACE ( 'NONE', ( #1903 ), #13919, .T. ) ;
#10220=AXIS2_PLACEMENT_3D ( 'NONE', #13283, #6674, #13437 ) ;
#10224=ORIENTED_EDGE ( 'NONE', *, *, #4059, .F. ) ;
#10240=CIRCLE ( 'NONE', #1360, 5.000000000000004441 ) ;
#10241=CARTESIAN_POINT ( 'NONE',  ( -68.68170757442787533, -83.66032599071911591, 33.00000000000002842 ) ) ;
#10255=EDGE_LOOP ( 'NONE', ( #6901, #7090, #8587, #3129, #2233, #3772, #11876, #10403 ) ) ;
#10263=FILL_AREA_STYLE_COLOUR ( '', #1699 ) ;
#10271=DIRECTION ( 'NONE',  ( 0.000000000000000000, 0.000000000000000000, -1.000000000000000000 ) ) ;
#10293=CARTESIAN_POINT ( 'NONE',  ( 0.000000000000000000, 189.5765550933606107, -37.00000000000003553 ) ) ;
#10296=EDGE_CURVE ( 'NONE', #1320, #5390, #12071, .T. ) ;
#10308=AXIS2_PLACEMENT_3D ( 'NONE', #11628, #1380, #12803 ) ;
#10319=VECTOR ( 'NONE', #3821, 1000.000000000000000 ) ;
#10326=LINE ( 'NONE', #3609, #6798 ) ;
#10333=FACE_BOUND ( 'NONE', #9978, .T. ) ;
#10336=EDGE_LOOP ( 'NONE', ( #8840, #14073, #9802, #613 ) ) ;
#10338=CARTESIAN_POINT ( 'NONE',  ( 139.9999999999996874, 189.5765550933606107, 47.99999999999998579 ) ) ;
#10341=EDGE_CURVE ( 'NONE', #4966, #11019, #2617, .T. ) ;
#10343=LINE ( 'NONE', #9312, #3134 ) ;
#10347=DIRECTION ( 'NONE',  ( -1.000000000000000000, -1.723842398015259277E-15, 0.000000000000000000 ) ) ;
#10357=ORIENTED_EDGE ( 'NONE', *, *, #2136, .T. ) ;
#10361=VERTEX_POINT ( 'NONE', #6860 ) ;
#10375=DIRECTION ( 'NONE',  ( -0.000000000000000000, 1.000000000000000000, -0.000000000000000000 ) ) ;
#10376=FACE_OUTER_BOUND ( 'NONE', #626, .T. ) ;
#10378=ORIENTED_EDGE ( 'NONE', *, *, #6373, .T. ) ;
#10403=ORIENTED_EDGE ( 'NONE', *, *, #10470, .T. ) ;
#10407=LINE ( 'NONE', #3759, #11706 ) ;
#10411=ADVANCED_FACE ( 'NONE', ( #1442 ), #1519, .F. ) ;
#10425=ORIENTED_EDGE ( 'NONE', *, *, #10201, .F. ) ;
#10440=ORIENTED_EDGE ( 'NONE', *, *, #10946, .F. ) ;
#10443=EDGE_CURVE ( 'NONE', #4578, #6602, #13535, .T. ) ;
#10451=DIRECTION ( 'NONE',  ( 0.000000000000000000, -1.000000000000000000, 0.000000000000000000 ) ) ;
#10456=LINE ( 'NONE', #12731, #9612 ) ;
#10459=EDGE_LOOP ( 'NONE', ( #7592, #12125 ) ) ;
#10467=ORIENTED_EDGE ( 'NONE', *, *, #12518, .F. ) ;
#10470=EDGE_CURVE ( 'NONE', #10731, #562, #9193, .T. ) ;
#10473=CIRCLE ( 'NONE', #10944, 5.000000000000004441 ) ;
#10479=DIRECTION ( 'NONE',  ( -1.000000000000000000, 1.892425610156517368E-16, 0.000000000000000000 ) ) ;
#10480=VERTEX_POINT ( 'NONE', #5679 ) ;
#10482=CARTESIAN_POINT ( 'NONE',  ( -68.68170757442807428, 29.57655509336051125, 33.00000000000002842 ) ) ;
#10498=VECTOR ( 'NONE', #2226, 1000.000000000000000 ) ;
#10499=ORIENTED_EDGE ( 'NONE', *, *, #2573, .F. ) ;
#10501=EDGE_CURVE ( 'NONE', #1523, #7848, #10517, .T. ) ;
#10513=( NAMED_UNIT ( * ) SI_UNIT ( $, .STERADIAN. ) SOLID_ANGLE_UNIT ( ) );
#10514=DIRECTION ( 'NONE',  ( 1.000000000000000000, 1.913084959030911013E-15, 0.000000000000000000 ) ) ;
#10517=LINE ( 'NONE', #6198, #4696 ) ;
#10524=CARTESIAN_POINT ( 'NONE',  ( -108.6817075744281027, 39.57655509336044730, 33.00000000000002842 ) ) ;
#10525=ORIENTED_EDGE ( 'NONE', *, *, #1189, .F. ) ;
#10539=EDGE_CURVE ( 'NONE', #7758, #8708, #10669, .T. ) ;
#10541=DIRECTION ( 'NONE',  ( 0.000000000000000000, 1.000000000000000000, 0.000000000000000000 ) ) ;
#10543=VERTEX_POINT ( 'NONE', #497 ) ;
#10547=CARTESIAN_POINT ( 'NONE',  ( -140.0000000000003411, 189.5765550933606107, -132.0000000000000000 ) ) ;
#10561=DIRECTION ( 'NONE',  ( -1.723842398015259277E-15, 1.000000000000000000, 0.000000000000000000 ) ) ;
#10568=VERTEX_POINT ( 'NONE', #8385 ) ;
#10574=EDGE_CURVE ( 'NONE', #13865, #768, #11608, .T. ) ;
#10575=ORIENTED_EDGE ( 'NONE', *, *, #10341, .T. ) ;
#10597=DIRECTION ( 'NONE',  ( -1.892425610156516875E-16, -1.000000000000000000, 0.000000000000000000 ) ) ;
#10603=VERTEX_POINT ( 'NONE', #1096 ) ;
#10609=DIRECTION ( 'NONE',  ( 6.608470384673545847E-17, -1.000000000000000000, 0.000000000000000000 ) ) ;
#10617=AXIS2_PLACEMENT_3D ( 'NONE', #11359, #3414, #1272 ) ;
#10628=ORIENTED_EDGE ( 'NONE', *, *, #12197, .T. ) ;
#10642=( LENGTH_UNIT ( ) NAMED_UNIT ( * ) SI_UNIT ( .MILLI., .METRE. ) );
#10650=LINE ( 'NONE', #8366, #5791 ) ;
#10652=VERTEX_POINT ( 'NONE', #7751 ) ;
#10660=ORIENTED_EDGE ( 'NONE', *, *, #3843, .F. ) ;
#10669=LINE ( 'NONE', #3870, #13829 ) ;
#10676=ORIENTED_EDGE ( 'NONE', *, *, #10443, .F. ) ;
#10690=EDGE_CURVE ( 'NONE', #5040, #10067, #5867, .T. ) ;
#10696=ORIENTED_EDGE ( 'NONE', *, *, #13134, .T. ) ;
#10702=EDGE_CURVE ( 'NONE', #9034, #1523, #1451, .T. ) ;
#10706=CARTESIAN_POINT ( 'NONE',  ( 129.3408537872138595, 199.5765550933606107, -75.00000000000001421 ) ) ;
#10726=EDGE_CURVE ( 'NONE', #1344, #11757, #3168, .T. ) ;
#10731=VERTEX_POINT ( 'NONE', #875 ) ;
#10797=ADVANCED_FACE ( 'NONE', ( #4756 ), #7962, .F. ) ;
#10835=DIRECTION ( 'NONE',  ( 0.000000000000000000, -1.000000000000000000, 0.000000000000000000 ) ) ;
#10846=VECTOR ( 'NONE', #1876, 1000.000000000000000 ) ;
#10855=EDGE_CURVE ( 'NONE', #254, #6531, #7004, .T. ) ;
#10867=ORIENTED_EDGE ( 'NONE', *, *, #1962, .F. ) ;
#10871=CARTESIAN_POINT ( 'NONE',  ( -118.6817075744281595, 69.57655509336025546, 0.000000000000000000 ) ) ;
#10874=CARTESIAN_POINT ( 'NONE',  ( 118.6817075744280316, 109.5765550933604828, -3.299999999999976730 ) ) ;
#10883=EDGE_LOOP ( 'NONE', ( #11053, #13160, #3808, #1895 ) ) ;
#10890=CARTESIAN_POINT ( 'NONE',  ( 129.3408537872138595, 189.5765550933606107, -9.000000000000007105 ) ) ;
#10898=AXIS2_PLACEMENT_3D ( 'NONE', #5358, #13433, #3328 ) ;
#10902=EDGE_CURVE ( 'NONE', #433, #13172, #3665, .T. ) ;
#10933=ORIENTED_EDGE ( 'NONE', *, *, #5871, .F. ) ;
#10944=AXIS2_PLACEMENT_3D ( 'NONE', #9714, #5035, #11990 ) ;
#10946=EDGE_CURVE ( 'NONE', #12513, #6374, #5047, .T. ) ;
#10959=DIRECTION ( 'NONE',  ( 0.000000000000000000, 0.000000000000000000, -1.000000000000000000 ) ) ;
#10976=EDGE_CURVE ( 'NONE', #10034, #10067, #668, .T. ) ;
#10985=DIRECTION ( 'NONE',  ( 0.000000000000000000, 0.000000000000000000, -1.000000000000000000 ) ) ;
#10994=PLANE ( 'NONE',  #3928 ) ;
#11001=CIRCLE ( 'NONE', #9837, 3.299999999999969624 ) ;
#11003=DIRECTION ( 'NONE',  ( -1.892425610156516875E-16, -1.000000000000000000, 0.000000000000000000 ) ) ;
#11014=EDGE_CURVE ( 'NONE', #4578, #3893, #11001, .T. ) ;
#11019=VERTEX_POINT ( 'NONE', #442 ) ;
#11025=AXIS2_PLACEMENT_3D ( 'NONE', #167, #6524, #5441 ) ;
#11026=ORIENTED_EDGE ( 'NONE', *, *, #8362, .T. ) ;
#11053=ORIENTED_EDGE ( 'NONE', *, *, #9049, .F. ) ;
#11066=EDGE_CURVE ( 'NONE', #4711, #5054, #11555, .T. ) ;
#11068=EDGE_CURVE ( 'NONE', #12928, #8708, #2562, .T. ) ;
#11069=AXIS2_PLACEMENT_3D ( 'NONE', #6204, #13906, #722 ) ;
#11073=CARTESIAN_POINT ( 'NONE',  ( 118.6817075744280316, 69.57655509336046862, 0.000000000000000000 ) ) ;
#11080=ORIENTED_EDGE ( 'NONE', *, *, #8871, .F. ) ;
#11086=CARTESIAN_POINT ( 'NONE',  ( -108.6817075744283869, 189.5765550933606107, 33.00000000000002842 ) ) ;
#11112=EDGE_LOOP ( 'NONE', ( #2730, #112 ) ) ;
#11116=AXIS2_PLACEMENT_3D ( 'NONE', #14157, #14227, #1259 ) ;
#11117=EDGE_LOOP ( 'NONE', ( #1769, #11169, #1097, #256 ) ) ;
#11127=EDGE_LOOP ( 'NONE', ( #3973, #3208, #5162, #12774 ) ) ;
#11128=CARTESIAN_POINT ( 'NONE',  ( 118.6817075744280316, 109.5765550933604828, 3.299999999999983391 ) ) ;
#11149=CARTESIAN_POINT ( 'NONE',  ( -118.6817075744281595, 69.57655509336025546, -3.299999999999983391 ) ) ;
#11157=DIRECTION ( 'NONE',  ( 0.000000000000000000, 1.000000000000000000, -0.000000000000000000 ) ) ;
#11169=ORIENTED_EDGE ( 'NONE', *, *, #8635, .T. ) ;
#11204=DIRECTION ( 'NONE',  ( 1.000000000000000000, 8.619211990076297369E-16, 0.000000000000000000 ) ) ;
#11212=LINE ( 'NONE', #8201, #6716 ) ;
#11216=LINE ( 'NONE', #2438, #4749 ) ;
#11219=CARTESIAN_POINT ( 'NONE',  ( 129.3408537872138595, 189.5765550933606107, -13.99999999999999645 ) ) ;
#11221=ADVANCED_FACE ( 'NONE', ( #12882 ), #1683, .F. ) ;
#11224=CARTESIAN_POINT ( 'NONE',  ( -68.68170757442808849, 39.57655509336051836, -106.9999999999999858 ) ) ;
#11232=CARTESIAN_POINT ( 'NONE',  ( -118.6817075744283727, 189.5765550933606107, 33.00000000000002842 ) ) ;
#11234=DIRECTION ( 'NONE',  ( -0.000000000000000000, 1.000000000000000000, -0.000000000000000000 ) ) ;
#11254=CARTESIAN_POINT ( 'NONE',  ( 0.000000000000000000, 0.000000000000000000, -117.0000000000000000 ) ) ;
#11259=ORIENTED_EDGE ( 'NONE', *, *, #10201, .T. ) ;
#11264=CARTESIAN_POINT ( 'NONE',  ( -140.0000000000003411, 199.5765550933606107, 47.99999999999998579 ) ) ;
#11277=CARTESIAN_POINT ( 'NONE',  ( -68.68170757442787533, -83.66032599071911591, -117.0000000000000000 ) ) ;
#11282=CIRCLE ( 'NONE', #7532, 3.299999999999969624 ) ;
#11289=APPLICATION_CONTEXT ( 'automotive_design' ) ;
#11297=EDGE_CURVE ( 'NONE', #1344, #2782, #731, .T. ) ;
#11298=DIRECTION ( 'NONE',  ( -1.000000000000000000, 0.000000000000000000, 1.387778780781446415E-16 ) ) ;
#11303=SURFACE_SIDE_STYLE ('',( #13446 ) ) ;
#11311=CYLINDRICAL_SURFACE ( 'NONE', #2747, 3.299999999999976730 ) ;
#11315=EDGE_LOOP ( 'NONE', ( #1993, #10017 ) ) ;
#11324=CARTESIAN_POINT ( 'NONE',  ( -118.6817075744279606, -30.42344490663958112, 33.00000000000002842 ) ) ;
#11359=CARTESIAN_POINT ( 'NONE',  ( 88.22284556172391490, 39.57655509336063915, -117.0000000000000000 ) ) ;
#11394=ORIENTED_EDGE ( 'NONE', *, *, #10946, .T. ) ;
#11399=AXIS2_PLACEMENT_3D ( 'NONE', #11766, #10514, #3940 ) ;
#11404=CARTESIAN_POINT ( 'NONE',  ( -108.6817075744279748, -20.42344490663957046, 33.00000000000002842 ) ) ;
#11409=( GEOMETRIC_REPRESENTATION_CONTEXT ( 3 ) GLOBAL_UNCERTAINTY_ASSIGNED_CONTEXT ( ( #4846 ) ) GLOBAL_UNIT_ASSIGNED_CONTEXT ( ( #6032, #8234, #10513 ) ) REPRESENTATION_CONTEXT ( 'NONE', 'WORKASPACE' ) );
#11413=CARTESIAN_POINT ( 'NONE',  ( 108.6817075744280316, -20.42344490663947809, -32.00000000000002842 ) ) ;
#11421=ORIENTED_EDGE ( 'NONE', *, *, #10726, .T. ) ;
#11440=ORIENTED_EDGE ( 'NONE', *, *, #14144, .F. ) ;
#11441=CARTESIAN_POINT ( 'NONE',  ( -108.6817075744280316, -20.42344490663947809, -32.00000000000002842 ) ) ;
#11450=AXIS2_PLACEMENT_3D ( 'NONE', #9389, #6080, #8577 ) ;
#11464=DIRECTION ( 'NONE',  ( -1.000000000000000000, 0.000000000000000000, 0.000000000000000000 ) ) ;
#11487=ORIENTED_EDGE ( 'NONE', *, *, #5036, .T. ) ;
#11511=SHAPE_REPRESENTATION_RELATIONSHIP ( 'NONE' , 'NONE' ,  #11805, #14323 ) ;
#11516=CARTESIAN_POINT ( 'NONE',  ( -129.3408537872145132, 189.5765550933606107, -9.000000000000007105 ) ) ;
#11517=LINE ( 'NONE', #6970, #2511 ) ;
#11526=CIRCLE ( 'NONE', #5214, 5.000000000000004441 ) ;
#11528=CARTESIAN_POINT ( 'NONE',  ( 118.6817075744280601, 189.5765550933606107, 33.00000000000002842 ) ) ;
#11533=SURFACE_STYLE_USAGE ( .BOTH. , #1659 ) ;
#11552=LINE ( 'NONE', #8318, #6519 ) ;
#11555=LINE ( 'NONE', #4823, #7021 ) ;
#11565=CARTESIAN_POINT ( 'NONE',  ( -108.6817075744279748, -20.42344490663957046, 33.00000000000002842 ) ) ;
#11568=EDGE_CURVE ( 'NONE', #10568, #7189, #3799, .T. ) ;
#11574=EDGE_LOOP ( 'NONE', ( #6491, #12437, #5306, #393, #7748, #11421, #13789, #12788 ) ) ;
#11577=LINE ( 'NONE', #6003, #9425 ) ;
#11608=LINE ( 'NONE', #13899, #500 ) ;
#11621=DIRECTION ( 'NONE',  ( 1.000000000000000000, 0.000000000000000000, 0.000000000000000000 ) ) ;
#11628=CARTESIAN_POINT ( 'NONE',  ( -129.3408537872145132, 189.5765550933606107, -9.000000000000007105 ) ) ;
#11640=ADVANCED_FACE ( 'NONE', ( #8602 ), #13090, .T. ) ;
#11657=FACE_OUTER_BOUND ( 'NONE', #7053, .T. ) ;
#11685=CARTESIAN_POINT ( 'NONE',  ( 24.99999999999998934, -30.42444490663959300, -2.000000000000001776 ) ) ;
#11689=EDGE_CURVE ( 'NONE', #12513, #13862, #2176, .T. ) ;
#11692=ORIENTED_EDGE ( 'NONE', *, *, #1189, .T. ) ;
#11706=VECTOR ( 'NONE', #7105, 1000.000000000000000 ) ;
#11733=AXIS2_PLACEMENT_3D ( 'NONE', #13864, #12522, #12590 ) ;
#11757=VERTEX_POINT ( 'NONE', #3566 ) ;
#11766=CARTESIAN_POINT ( 'NONE',  ( -108.6817075744279748, -20.42344490663957046, 33.00000000000002842 ) ) ;
#11777=DIRECTION ( 'NONE',  ( 1.000000000000000000, -0.000000000000000000, 0.000000000000000000 ) ) ;
#11789=CARTESIAN_POINT ( 'NONE',  ( 129.3408537872138595, 189.5765550933606107, -75.00000000000001421 ) ) ;
#11804=ORIENTED_EDGE ( 'NONE', *, *, #10855, .F. ) ;
#11805=SHAPE_REPRESENTATION ( 'Cast Steel Wedge Housing Block', ( #11025 ), #532 ) ;
#11819=FACE_OUTER_BOUND ( 'NONE', #2967, .T. ) ;
#11833=ADVANCED_FACE ( 'NONE', ( #9170 ), #8139, .T. ) ;
#11840=EDGE_CURVE ( 'NONE', #10361, #3683, #9838, .T. ) ;
#11861=ORIENTED_EDGE ( 'NONE', *, *, #6864, .F. ) ;
#11876=ORIENTED_EDGE ( 'NONE', *, *, #8635, .F. ) ;
#11896=VERTEX_POINT ( 'NONE', #2674 ) ;
#11903=ORIENTED_EDGE ( 'NONE', *, *, #10574, .T. ) ;
#11930=LINE ( 'NONE', #8556, #6585 ) ;
#11932=VERTEX_POINT ( 'NONE', #5229 ) ;
#11944=ORIENTED_EDGE ( 'NONE', *, *, #7072, .T. ) ;
#11946=EDGE_CURVE ( 'NONE', #11896, #7758, #6244, .T. ) ;
#11959=AXIS2_PLACEMENT_3D ( 'NONE', #9796, #8405, #9587 ) ;
#11974=VECTOR ( 'NONE', #7100, 1000.000000000000000 ) ;
#11979=ORIENTED_EDGE ( 'NONE', *, *, #7524, .F. ) ;
#11982=LINE ( 'NONE', #1958, #4638 ) ;
#11987=DIRECTION ( 'NONE',  ( 0.000000000000000000, -1.000000000000000000, 0.000000000000000000 ) ) ;
#11990=DIRECTION ( 'NONE',  ( 0.000000000000000000, 0.000000000000000000, -1.000000000000000000 ) ) ;
#11999=DIRECTION ( 'NONE',  ( -1.000000000000000000, -0.000000000000000000, 1.387778780781446169E-16 ) ) ;
#12023=LINE ( 'NONE', #5594, #1818 ) ;
#12025=DIRECTION ( 'NONE',  ( -1.000000000000000000, -1.913084959030911013E-15, -0.000000000000000000 ) ) ;
#12032=EDGE_CURVE ( 'NONE', #3683, #6291, #1308, .T. ) ;
#12034=CARTESIAN_POINT ( 'NONE',  ( 129.3408537872138595, 189.5765550933606107, -80.00000000000002842 ) ) ;
#12041=DIRECTION ( 'NONE',  ( 1.000000000000000000, 0.000000000000000000, 0.000000000000000000 ) ) ;
#12059=ORIENTED_EDGE ( 'NONE', *, *, #5959, .T. ) ;
#12071=LINE ( 'NONE', #8836, #13385 ) ;
#12084=ORIENTED_EDGE ( 'NONE', *, *, #4165, .F. ) ;
#12089=ORIENTED_EDGE ( 'NONE', *, *, #7163, .F. ) ;
#12100=CIRCLE ( 'NONE', #7638, 3.299999999999983391 ) ;
#12104=ORIENTED_EDGE ( 'NONE', *, *, #10539, .F. ) ;
#12105=DIRECTION ( 'NONE',  ( 0.000000000000000000, 0.000000000000000000, -1.000000000000000000 ) ) ;
#12113=CARTESIAN_POINT ( 'NONE',  ( -24.99999999999998934, 189.5765550933606107, -2.000000000000001776 ) ) ;
#12117=CARTESIAN_POINT ( 'NONE',  ( 118.6817075744280316, 69.57655509336046862, 0.000000000000000000 ) ) ;
#12125=ORIENTED_EDGE ( 'NONE', *, *, #12379, .F. ) ;
#12148=DIRECTION ( 'NONE',  ( 0.000000000000000000, -1.000000000000000000, 0.000000000000000000 ) ) ;
#12154=CARTESIAN_POINT ( 'NONE',  ( 118.6817075744280316, 69.57655509336046862, 0.000000000000000000 ) ) ;
#12164=CARTESIAN_POINT ( 'NONE',  ( 108.6817075744280316, 39.57655509336063915, 33.00000000000002842 ) ) ;
#12169=CYLINDRICAL_SURFACE ( 'NONE', #12196, 4.999999999999976907 ) ;
#12175=EDGE_CURVE ( 'NONE', #1477, #2782, #2719, .T. ) ;
#12177=DIRECTION ( 'NONE',  ( -2.081668171172168760E-16, 0.000000000000000000, -1.000000000000000000 ) ) ;
#12185=CARTESIAN_POINT ( 'NONE',  ( -108.6817075744279748, -20.42344490663957046, -106.9999999999999858 ) ) ;
#12195=AXIS2_PLACEMENT_3D ( 'NONE', #10293, #10375, #12562 ) ;
#12196=AXIS2_PLACEMENT_3D ( 'NONE', #5506, #9659, #6214 ) ;
#12197=EDGE_CURVE ( 'NONE', #5014, #13727, #9362, .T. ) ;
#12216=VERTEX_POINT ( 'NONE', #7152 ) ;
#12218=EDGE_CURVE ( 'NONE', #6374, #12928, #10456, .T. ) ;
#12229=EDGE_CURVE ( 'NONE', #3683, #10361, #8682, .T. ) ;
#12230=DIRECTION ( 'NONE',  ( 0.000000000000000000, -1.000000000000000000, 0.000000000000000000 ) ) ;
#12237=VERTEX_POINT ( 'NONE', #8327 ) ;
#12240=CARTESIAN_POINT ( 'NONE',  ( 0.000000000000000000, 199.5765550933606107, -37.00000000000003553 ) ) ;
#12255=AXIS2_PLACEMENT_3D ( 'NONE', #412, #12772, #1510 ) ;
#12264=EDGE_CURVE ( 'NONE', #1477, #2687, #1686, .T. ) ;
#12269=ORIENTED_EDGE ( 'NONE', *, *, #5255, .F. ) ;
#12282=DIRECTION ( 'NONE',  ( 0.000000000000000000, 1.000000000000000000, 0.000000000000000000 ) ) ;
#12298=CARTESIAN_POINT ( 'NONE',  ( 108.6817075744280316, 69.57655509336046862, 3.299999999999976730 ) ) ;
#12323=EDGE_CURVE ( 'NONE', #1219, #1, #12641, .T. ) ;
#12326=PRODUCT ( 'Cast Steel Wedge Housing Block', 'Cast Steel Wedge Housing Block', '', ( #4261 ) ) ;
#12332=LINE ( 'NONE', #14459, #9104 ) ;
#12347=ORIENTED_EDGE ( 'NONE', *, *, #12323, .T. ) ;
#12364=VECTOR ( 'NONE', #2410, 1000.000000000000000 ) ;
#12371=DIRECTION ( 'NONE',  ( 0.000000000000000000, 1.000000000000000000, 0.000000000000000000 ) ) ;
#12379=EDGE_CURVE ( 'NONE', #6291, #10652, #1914, .T. ) ;
#12396=DIRECTION ( 'NONE',  ( 1.734723475976807094E-16, 0.000000000000000000, -1.000000000000000000 ) ) ;
#12400=AXIS2_PLACEMENT_3D ( 'NONE', #11073, #3403, #6743 ) ;
#12416=EDGE_LOOP ( 'NONE', ( #6087, #11080, #7999, #9302 ) ) ;
#12422=VECTOR ( 'NONE', #5624, 1000.000000000000000 ) ;
#12437=ORIENTED_EDGE ( 'NONE', *, *, #4059, .T. ) ;
#12439=CARTESIAN_POINT ( 'NONE',  ( -24.99999999999998934, 199.5765550933606107, -2.000000000000001776 ) ) ;
#12441=ORIENTED_EDGE ( 'NONE', *, *, #3346, .T. ) ;
#12452=ORIENTED_EDGE ( 'NONE', *, *, #4034, .T. ) ;
#12454=VECTOR ( 'NONE', #4155, 1000.000000000000000 ) ;
#12468=DIRECTION ( 'NONE',  ( -1.387778780781446415E-16, 0.000000000000000000, -1.000000000000000000 ) ) ;
#12479=EDGE_LOOP ( 'NONE', ( #2878, #7386 ) ) ;
#12498=PLANE ( 'NONE',  #7744 ) ;
#12512=LINE ( 'NONE', #10241, #1930 ) ;
#12513=VERTEX_POINT ( 'NONE', #11324 ) ;
#12518=EDGE_CURVE ( 'NONE', #11932, #10034, #6347, .T. ) ;
#12522=DIRECTION ( 'NONE',  ( -1.000000000000000000, 0.000000000000000000, 0.000000000000000000 ) ) ;
#12525=EDGE_CURVE ( 'NONE', #7201, #12696, #3654, .T. ) ;
#12530=DIRECTION ( 'NONE',  ( 0.000000000000000000, 0.000000000000000000, -1.000000000000000000 ) ) ;
#12540=DIRECTION ( 'NONE',  ( 0.000000000000000000, 1.000000000000000000, -0.000000000000000000 ) ) ;
#12558=DIRECTION ( 'NONE',  ( 1.000000000000000000, 0.000000000000000000, -0.000000000000000000 ) ) ;
#12561=ADVANCED_FACE ( 'NONE', ( #9343 ), #12498, .T. ) ;
#12562=DIRECTION ( 'NONE',  ( 0.000000000000000000, 0.000000000000000000, -1.000000000000000000 ) ) ;
#12583=LINE ( 'NONE', #12658, #3677 ) ;
#12590=DIRECTION ( 'NONE',  ( 0.000000000000000000, 0.000000000000000000, 1.000000000000000000 ) ) ;
#12606=ADVANCED_FACE ( 'NONE', ( #6116, #1667, #8387 ), #582, .T. ) ;
#12610=CARTESIAN_POINT ( 'NONE',  ( -129.3408537872145132, 189.5765550933606107, -75.00000000000001421 ) ) ;
#12612=ORIENTED_EDGE ( 'NONE', *, *, #5959, .F. ) ;
#12615=AXIS2_PLACEMENT_3D ( 'NONE', #7494, #11987, #1963 ) ;
#12623=LINE ( 'NONE', #4808, #4878 ) ;
#12634=DIRECTION ( 'NONE',  ( 0.000000000000000000, 0.000000000000000000, -1.000000000000000000 ) ) ;
#12636=ADVANCED_FACE ( 'NONE', ( #6802 ), #5627, .F. ) ;
#12641=CIRCLE ( 'NONE', #13371, 5.000000000000018652 ) ;
#12646=DIRECTION ( 'NONE',  ( -1.913084959030911013E-15, 1.000000000000000000, 0.000000000000000000 ) ) ;
#12647=DIRECTION ( 'NONE',  ( -2.081668171172169006E-16, -0.000000000000000000, 1.000000000000000000 ) ) ;
#12651=ORIENTED_EDGE ( 'NONE', *, *, #11297, .T. ) ;
#12653=AXIS2_PLACEMENT_3D ( 'NONE', #8441, #12924, #7342 ) ;
#12658=CARTESIAN_POINT ( 'NONE',  ( 0.000000000000000000, 189.5765550933606107, 33.00000000000002842 ) ) ;
#12674=ADVANCED_FACE ( 'NONE', ( #5693 ), #7753, .F. ) ;
#12679=FACE_BOUND ( 'NONE', #14449, .T. ) ;
#12683=VECTOR ( 'NONE', #9399, 1000.000000000000000 ) ;
#12696=VERTEX_POINT ( 'NONE', #5489 ) ;
#12722=CARTESIAN_POINT ( 'NONE',  ( -140.0000000000003411, 189.5765550933606107, 47.99999999999998579 ) ) ;
#12723=PLANE ( 'NONE',  #9833 ) ;
#12731=CARTESIAN_POINT ( 'NONE',  ( -118.6817075744279748, -20.42344490663959178, -117.0000000000000000 ) ) ;
#12734=ORIENTED_EDGE ( 'NONE', *, *, #11689, .T. ) ;
#12736=ORIENTED_EDGE ( 'NONE', *, *, #898, .T. ) ;
#12754=FACE_BOUND ( 'NONE', #2335, .T. ) ;
#12755=( NAMED_UNIT ( * ) PLANE_ANGLE_UNIT ( ) SI_UNIT ( $, .RADIAN. ) );
#12763=ADVANCED_FACE ( 'NONE', ( #4347, #2502, #5777 ), #9230, .F. ) ;
#12765=ORIENTED_EDGE ( 'NONE', *, *, #5991, .F. ) ;
#12772=DIRECTION ( 'NONE',  ( 0.000000000000000000, 0.000000000000000000, 1.000000000000000000 ) ) ;
#12774=ORIENTED_EDGE ( 'NONE', *, *, #2464, .F. ) ;
#12780=DIRECTION ( 'NONE',  ( 1.892425610156517122E-16, 1.000000000000000000, 0.000000000000000000 ) ) ;
#12788=ORIENTED_EDGE ( 'NONE', *, *, #2070, .T. ) ;
#12795=DIRECTION ( 'NONE',  ( -1.913084959030911013E-15, 1.000000000000000000, 0.000000000000000000 ) ) ;
#12796=AXIS2_PLACEMENT_3D ( 'NONE', #9477, #1643, #3051 ) ;
#12803=DIRECTION ( 'NONE',  ( 0.000000000000000000, 0.000000000000000000, 1.000000000000000000 ) ) ;
#12819=AXIS2_PLACEMENT_3D ( 'NONE', #82, #4556, #12148 ) ;
#12821=EDGE_CURVE ( 'NONE', #7848, #6549, #3796, .T. ) ;
#12825=CARTESIAN_POINT ( 'NONE',  ( 118.6817075744280174, -30.42344490663937506, -117.0000000000000000 ) ) ;
#12844=DIRECTION ( 'NONE',  ( -1.000000000000000000, -1.723842398015259277E-15, 0.000000000000000000 ) ) ;
#12856=ADVANCED_FACE ( 'NONE', ( #537 ), #3754, .T. ) ;
#12875=EDGE_CURVE ( 'NONE', #13737, #9480, #1397, .T. ) ;
#12877=CARTESIAN_POINT ( 'NONE',  ( -108.6817075744279890, 189.5765550933605823, -106.9999999999999858 ) ) ;
#12881=ORIENTED_EDGE ( 'NONE', *, *, #6925, .F. ) ;
#12882=FACE_OUTER_BOUND ( 'NONE', #4509, .T. ) ;
#12924=DIRECTION ( 'NONE',  ( 1.723842398015259277E-15, -1.000000000000000000, 0.000000000000000000 ) ) ;
#12928=VERTEX_POINT ( 'NONE', #9602 ) ;
#12966=DIRECTION ( 'NONE',  ( 0.000000000000000000, 0.000000000000000000, 1.000000000000000000 ) ) ;
#12968=LINE ( 'NONE', #14134, #3053 ) ;
#13006=ORIENTED_EDGE ( 'NONE', *, *, #13970, .F. ) ;
#13030=CARTESIAN_POINT ( 'NONE',  ( -118.6817075744282306, 109.5765550933602697, 0.000000000000000000 ) ) ;
#13041=DIRECTION ( 'NONE',  ( 0.000000000000000000, 0.000000000000000000, 1.000000000000000000 ) ) ;
#13052=CARTESIAN_POINT ( 'NONE',  ( -140.0000000000003411, 189.5765550933606107, 47.99999999999998579 ) ) ;
#13058=UNCERTAINTY_MEASURE_WITH_UNIT (LENGTH_MEASURE( 1.000000000000000082E-05 ), #10642, 'distance_accuracy_value', 'NONE');
#13090=PLANE ( 'NONE',  #12615 ) ;
#13122=VECTOR ( 'NONE', #1132, 1000.000000000000000 ) ;
#13129=ORIENTED_EDGE ( 'NONE', *, *, #11068, .T. ) ;
#13134=EDGE_CURVE ( 'NONE', #13727, #14013, #12512, .T. ) ;
#13146=CARTESIAN_POINT ( 'NONE',  ( 68.68170757442801744, 39.57655509336063915, -106.9999999999999858 ) ) ;
#13160=ORIENTED_EDGE ( 'NONE', *, *, #999, .T. ) ;
#13172=VERTEX_POINT ( 'NONE', #1536 ) ;
#13195=CARTESIAN_POINT ( 'NONE',  ( 88.22284556172391490, 39.57655509336063915, 33.00000000000002842 ) ) ;
#13204=CARTESIAN_POINT ( 'NONE',  ( -108.6817075744281595, 69.57655509336026967, 3.299999999999976730 ) ) ;
#13205=CARTESIAN_POINT ( 'NONE',  ( -108.6817075744282448, 109.5765550933602839, 0.000000000000000000 ) ) ;
#13206=DIRECTION ( 'NONE',  ( 0.000000000000000000, 0.000000000000000000, 1.000000000000000000 ) ) ;
#13217=ORIENTED_EDGE ( 'NONE', *, *, #6206, .T. ) ;
#13238=ORIENTED_EDGE ( 'NONE', *, *, #4255, .T. ) ;
#13239=DIRECTION ( 'NONE',  ( 0.000000000000000000, 0.000000000000000000, 1.000000000000000000 ) ) ;
#13260=DIRECTION ( 'NONE',  ( 0.000000000000000000, 1.000000000000000000, 0.000000000000000000 ) ) ;
#13267=DIRECTION ( 'NONE',  ( 0.000000000000000000, 0.000000000000000000, 1.000000000000000000 ) ) ;
#13269=VECTOR ( 'NONE', #5385, 1000.000000000000000 ) ;
#13276=PLANE ( 'NONE',  #8868 ) ;
#13283=CARTESIAN_POINT ( 'NONE',  ( -2.501150643247835315E-15, -20.42344490663947809, 33.00000000000002842 ) ) ;
#13298=DIRECTION ( 'NONE',  ( 1.000000000000000000, -0.000000000000000000, -0.000000000000000000 ) ) ;
#13314=VECTOR ( 'NONE', #11621, 1000.000000000000000 ) ;
#13316=DIRECTION ( 'NONE',  ( -0.000000000000000000, -0.000000000000000000, 1.000000000000000000 ) ) ;
#13338=CARTESIAN_POINT ( 'NONE',  ( 118.6817075744280174, -30.42344490663937506, 33.00000000000002842 ) ) ;
#13346=CIRCLE ( 'NONE', #12400, 3.299999999999983391 ) ;
#13348=CARTESIAN_POINT ( 'NONE',  ( 108.6817075744280459, 189.5765550933606107, -106.9999999999999858 ) ) ;
#13352=ADVANCED_FACE ( 'NONE', ( #14069 ), #675, .F. ) ;
#13371=AXIS2_PLACEMENT_3D ( 'NONE', #11789, #5333, #3019 ) ;
#13385=VECTOR ( 'NONE', #13316, 1000.000000000000000 ) ;
#13387=EDGE_LOOP ( 'NONE', ( #8191, #4087, #12441, #11259 ) ) ;
#13388=ORIENTED_EDGE ( 'NONE', *, *, #7881, .T. ) ;
#13414=DIRECTION ( 'NONE',  ( -1.000000000000000000, 1.892425610156516875E-16, 0.000000000000000000 ) ) ;
#13433=DIRECTION ( 'NONE',  ( 1.000000000000000000, -0.000000000000000000, -0.000000000000000000 ) ) ;
#13437=DIRECTION ( 'NONE',  ( -1.000000000000000000, -8.619211990076296383E-16, 0.000000000000000000 ) ) ;
#13444=DIRECTION ( 'NONE',  ( 0.000000000000000000, 1.000000000000000000, 0.000000000000000000 ) ) ;
#13446=SURFACE_STYLE_FILL_AREA ( #9241 ) ;
#13450=EDGE_CURVE ( 'NONE', #3640, #10543, #3577, .T. ) ;
#13452=DIRECTION ( 'NONE',  ( 0.000000000000000000, 0.000000000000000000, -1.000000000000000000 ) ) ;
#13459=EDGE_LOOP ( 'NONE', ( #9501, #3679, #13217, #597 ) ) ;
#13472=DIRECTION ( 'NONE',  ( 1.000000000000000000, -0.000000000000000000, -0.000000000000000000 ) ) ;
#13490=ORIENTED_EDGE ( 'NONE', *, *, #12218, .F. ) ;
#13499=CARTESIAN_POINT ( 'NONE',  ( 0.000000000000000000, -30.42444490663959300, -37.00000000000003553 ) ) ;
#13509=CARTESIAN_POINT ( 'NONE',  ( -140.0000000000003411, 199.5765550933606107, -132.0000000000000000 ) ) ;
#13510=CARTESIAN_POINT ( 'NONE',  ( -108.6817075744279890, 189.5765550933605823, -106.9999999999999858 ) ) ;
#13519=CIRCLE ( 'NONE', #4851, 4.999999999999988454 ) ;
#13535=LINE ( 'NONE', #5961, #14062 ) ;
#13555=ORIENTED_EDGE ( 'NONE', *, *, #12821, .F. ) ;
#13557=ORIENTED_EDGE ( 'NONE', *, *, #1469, .F. ) ;
#13563=EDGE_CURVE ( 'NONE', #3893, #4578, #11282, .T. ) ;
#13576=ORIENTED_EDGE ( 'NONE', *, *, #6576, .T. ) ;
#13582=CARTESIAN_POINT ( 'NONE',  ( 139.9999999999996874, 189.5765550933606107, -132.0000000000000000 ) ) ;
#13584=( LENGTH_UNIT ( ) NAMED_UNIT ( * ) SI_UNIT ( .MILLI., .METRE. ) );
#13586=DIRECTION ( 'NONE',  ( 1.000000000000000000, 1.276920294826118092E-16, -0.000000000000000000 ) ) ;
#13592=VECTOR ( 'NONE', #10166, 1000.000000000000000 ) ;
#13595=ORIENTED_EDGE ( 'NONE', *, *, #13970, .T. ) ;
#13599=EDGE_LOOP ( 'NONE', ( #8513, #11979, #6475, #6331, #6658, #7408 ) ) ;
#13632=CARTESIAN_POINT ( 'NONE',  ( 108.6817075744280601, 189.5765550933606107, 33.00000000000002842 ) ) ;
#13634=VECTOR ( 'NONE', #9524, 1000.000000000000000 ) ;
#13642=VECTOR ( 'NONE', #8222, 1000.000000000000000 ) ;
#13643=DIRECTION ( 'NONE',  ( 1.913084959030911013E-15, -1.000000000000000000, 0.000000000000000000 ) ) ;
#13645=EDGE_CURVE ( 'NONE', #12237, #5054, #13811, .T. ) ;
#13649=FACE_OUTER_BOUND ( 'NONE', #7807, .T. ) ;
#13657=DIRECTION ( 'NONE',  ( 0.000000000000000000, 1.000000000000000000, 0.000000000000000000 ) ) ;
#13662=FACE_BOUND ( 'NONE', #11315, .T. ) ;
#13664=CARTESIAN_POINT ( 'NONE',  ( 108.6817075744280743, -20.42344490663954204, -106.9999999999999858 ) ) ;
#13666=DIRECTION ( 'NONE',  ( 0.000000000000000000, 1.000000000000000000, 0.000000000000000000 ) ) ;
#13681=EDGE_CURVE ( 'NONE', #3463, #11019, #977, .T. ) ;
#13690=ORIENTED_EDGE ( 'NONE', *, *, #10902, .T. ) ;
#13698=CARTESIAN_POINT ( 'NONE',  ( 0.000000000000000000, 189.5765550933606107, -117.0000000000000000 ) ) ;
#13704=CIRCLE ( 'NONE', #4134, 5.000000000000018652 ) ;
#13707=EDGE_CURVE ( 'NONE', #6374, #7758, #779, .T. ) ;
#13720=DIRECTION ( 'NONE',  ( 0.000000000000000000, 0.000000000000000000, -1.000000000000000000 ) ) ;
#13727=VERTEX_POINT ( 'NONE', #835 ) ;
#13735=ORIENTED_EDGE ( 'NONE', *, *, #6968, .F. ) ;
#13737=VERTEX_POINT ( 'NONE', #4225 ) ;
#13742=ORIENTED_EDGE ( 'NONE', *, *, #2065, .T. ) ;
#13755=ORIENTED_EDGE ( 'NONE', *, *, #10702, .F. ) ;
#13761=ORIENTED_EDGE ( 'NONE', *, *, #11689, .F. ) ;
#13785=EDGE_CURVE ( 'NONE', #11019, #6031, #11216, .T. ) ;
#13789=ORIENTED_EDGE ( 'NONE', *, *, #14144, .T. ) ;
#13811=LINE ( 'NONE', #3779, #13642 ) ;
#13814=ORIENTED_EDGE ( 'NONE', *, *, #7993, .F. ) ;
#13829=VECTOR ( 'NONE', #12780, 1000.000000000000000 ) ;
#13862=VERTEX_POINT ( 'NONE', #9981 ) ;
#13864=CARTESIAN_POINT ( 'NONE',  ( -140.0000000000003411, 189.5765550933606107, 47.99999999999998579 ) ) ;
#13865=VERTEX_POINT ( 'NONE', #4582 ) ;
#13875=AXIS2_PLACEMENT_3D ( 'NONE', #468, #8208, #13720 ) ;
#13899=CARTESIAN_POINT ( 'NONE',  ( 108.6817075744280459, 189.5765550933606107, -106.9999999999999858 ) ) ;
#13906=DIRECTION ( 'NONE',  ( -0.000000000000000000, 1.000000000000000000, -0.000000000000000000 ) ) ;
#13915=EDGE_LOOP ( 'NONE', ( #9861, #4703, #6365, #11440 ) ) ;
#13919=PLANE ( 'NONE',  #14081 ) ;
#13935=CARTESIAN_POINT ( 'NONE',  ( 108.6817075744280316, 69.57655509336046862, -3.299999999999976730 ) ) ;
#13945=ORIENTED_EDGE ( 'NONE', *, *, #3843, .T. ) ;
#13966=DIRECTION ( 'NONE',  ( -1.000000000000000000, 1.892425610156516875E-16, 0.000000000000000000 ) ) ;
#13970=EDGE_CURVE ( 'NONE', #3697, #3920, #1943, .T. ) ;
#13981=CARTESIAN_POINT ( 'NONE',  ( 129.3408537872138595, 199.5765550933606107, -75.00000000000001421 ) ) ;
#13998=ORIENTED_EDGE ( 'NONE', *, *, #7378, .T. ) ;
#14001=EDGE_CURVE ( 'NONE', #3393, #4966, #9232, .T. ) ;
#14013=VERTEX_POINT ( 'NONE', #10482 ) ;
#14022=ORIENTED_EDGE ( 'NONE', *, *, #5871, .T. ) ;
#14026=FACE_OUTER_BOUND ( 'NONE', #13387, .T. ) ;
#14046=DIRECTION ( 'NONE',  ( 1.000000000000000000, 1.723842398015259277E-15, -0.000000000000000000 ) ) ;
#14056=FACE_OUTER_BOUND ( 'NONE', #8853, .T. ) ;
#14062=VECTOR ( 'NONE', #6920, 1000.000000000000000 ) ;
#14065=DIRECTION ( 'NONE',  ( 1.892425610156516875E-16, 1.000000000000000000, 0.000000000000000000 ) ) ;
#14069=FACE_OUTER_BOUND ( 'NONE', #5480, .T. ) ;
#14073=ORIENTED_EDGE ( 'NONE', *, *, #10341, .F. ) ;
#14079=ORIENTED_EDGE ( 'NONE', *, *, #12264, .T. ) ;
#14081=AXIS2_PLACEMENT_3D ( 'NONE', #6056, #2794, #4975 ) ;
#14096=FACE_BOUND ( 'NONE', #481, .T. ) ;
#14131=FACE_OUTER_BOUND ( 'NONE', #10883, .T. ) ;
#14134=CARTESIAN_POINT ( 'NONE',  ( -24.99999999999998934, 199.5765550933606107, -2.000000000000001776 ) ) ;
#14135=CARTESIAN_POINT ( 'NONE',  ( 108.6817075744280316, 69.57655509336046862, 0.000000000000000000 ) ) ;
#14144=EDGE_CURVE ( 'NONE', #11757, #9480, #8718, .T. ) ;
#14150=ORIENTED_EDGE ( 'NONE', *, *, #11068, .F. ) ;
#14157=CARTESIAN_POINT ( 'NONE',  ( 129.3408537872138595, 189.5765550933606107, -75.00000000000001421 ) ) ;
#14169=DIRECTION ( 'NONE',  ( 1.000000000000000000, 1.723842398015259277E-15, -0.000000000000000000 ) ) ;
#14177=ORIENTED_EDGE ( 'NONE', *, *, #7642, .T. ) ;
#14184=CARTESIAN_POINT ( 'NONE',  ( -118.6817075744282306, 109.5765550933602697, 0.000000000000000000 ) ) ;
#14188=EDGE_CURVE ( 'NONE', #10067, #5040, #11526, .T. ) ;
#14209=ORIENTED_EDGE ( 'NONE', *, *, #5216, .T. ) ;
#14212=ORIENTED_EDGE ( 'NONE', *, *, #784, .F. ) ;
#14227=DIRECTION ( 'NONE',  ( 0.000000000000000000, 1.000000000000000000, 0.000000000000000000 ) ) ;
#14231=LINE ( 'NONE', #10040, #7952 ) ;
#14238=ORIENTED_EDGE ( 'NONE', *, *, #10726, .F. ) ;
#14241=CIRCLE ( 'NONE', #12819, 3.299999999999969624 ) ;
#14254=CIRCLE ( 'NONE', #4899, 5.000000000000018652 ) ;
#14276=ORIENTED_EDGE ( 'NONE', *, *, #7534, .F. ) ;
#14284=CIRCLE ( 'NONE', #7724, 3.299999999999969624 ) ;
#14285=DIRECTION ( 'NONE',  ( 0.000000000000000000, 1.000000000000000000, 0.000000000000000000 ) ) ;
#14287=EDGE_CURVE ( 'NONE', #10480, #3697, #334, .T. ) ;
#14296=EDGE_CURVE ( 'NONE', #10543, #3640, #6379, .T. ) ;
#14297=CARTESIAN_POINT ( 'NONE',  ( -118.6817075744282306, 109.5765550933602697, -3.299999999999976730 ) ) ;
#14298=CARTESIAN_POINT ( 'NONE',  ( 6.118061346828462449E-15, -30.42344490663947809, 33.00000000000002842 ) ) ;
#14310=LINE ( 'NONE', #7557, #6461 ) ;
#14318=CARTESIAN_POINT ( 'NONE',  ( -140.0000000000003411, 189.5765550933606107, 47.99999999999998579 ) ) ;
#14321=CARTESIAN_POINT ( 'NONE',  ( 108.6817075744280174, 39.57655509336063915, -117.0000000000000000 ) ) ;
#14323=ADVANCED_BREP_SHAPE_REPRESENTATION ( '', ( #6797, #11025 ), #532 ) ;
#14336=EDGE_LOOP ( 'NONE', ( #6015, #10051, #13742, #13945 ) ) ;
#14337=CARTESIAN_POINT ( 'NONE',  ( 108.6817075744280601, 39.57655509336063915, -106.9999999999999858 ) ) ;
#14347=ORIENTED_EDGE ( 'NONE', *, *, #14287, .T. ) ;
#14361=VECTOR ( 'NONE', #13657, 1000.000000000000000 ) ;
#14370=CARTESIAN_POINT ( 'NONE',  ( 108.6817075744280459, 109.5765550933604828, 3.299999999999976730 ) ) ;
#14372=DIRECTION ( 'NONE',  ( -1.000000000000000000, -8.619211990076296383E-16, 1.276920294826117846E-16 ) ) ;
#14392=DIRECTION ( 'NONE',  ( 0.000000000000000000, 1.000000000000000000, 0.000000000000000000 ) ) ;
#14394=DIRECTION ( 'NONE',  ( 1.000000000000000000, 1.723842398015259277E-15, 0.000000000000000000 ) ) ;
#14398=DIRECTION ( 'NONE',  ( 0.000000000000000000, 0.000000000000000000, -1.000000000000000000 ) ) ;
#14406=CARTESIAN_POINT ( 'NONE',  ( -140.0000000000003411, 199.5765550933606107, 47.99999999999998579 ) ) ;
#14408=LINE ( 'NONE', #3502, #4678 ) ;
#14422=LINE ( 'NONE', #11264, #12364 ) ;
#14432=AXIS2_PLACEMENT_3D ( 'NONE', #7837, #6515, #13206 ) ;
#14436=CARTESIAN_POINT ( 'NONE',  ( -108.6817075744282448, 109.5765550933602839, 0.000000000000000000 ) ) ;
#14449=EDGE_LOOP ( 'NONE', ( #692, #12084 ) ) ;
#14451=VERTEX_POINT ( 'NONE', #636 ) ;
#14457=CARTESIAN_POINT ( 'NONE',  ( 129.3408537872138595, 199.5765550933606107, -4.000000000000019540 ) ) ;
#14459=CARTESIAN_POINT ( 'NONE',  ( -129.3408537872145132, 189.5765550933606107, -4.000000000000031086 ) ) ;
ENDSEC;
END-ISO-10303-21;
